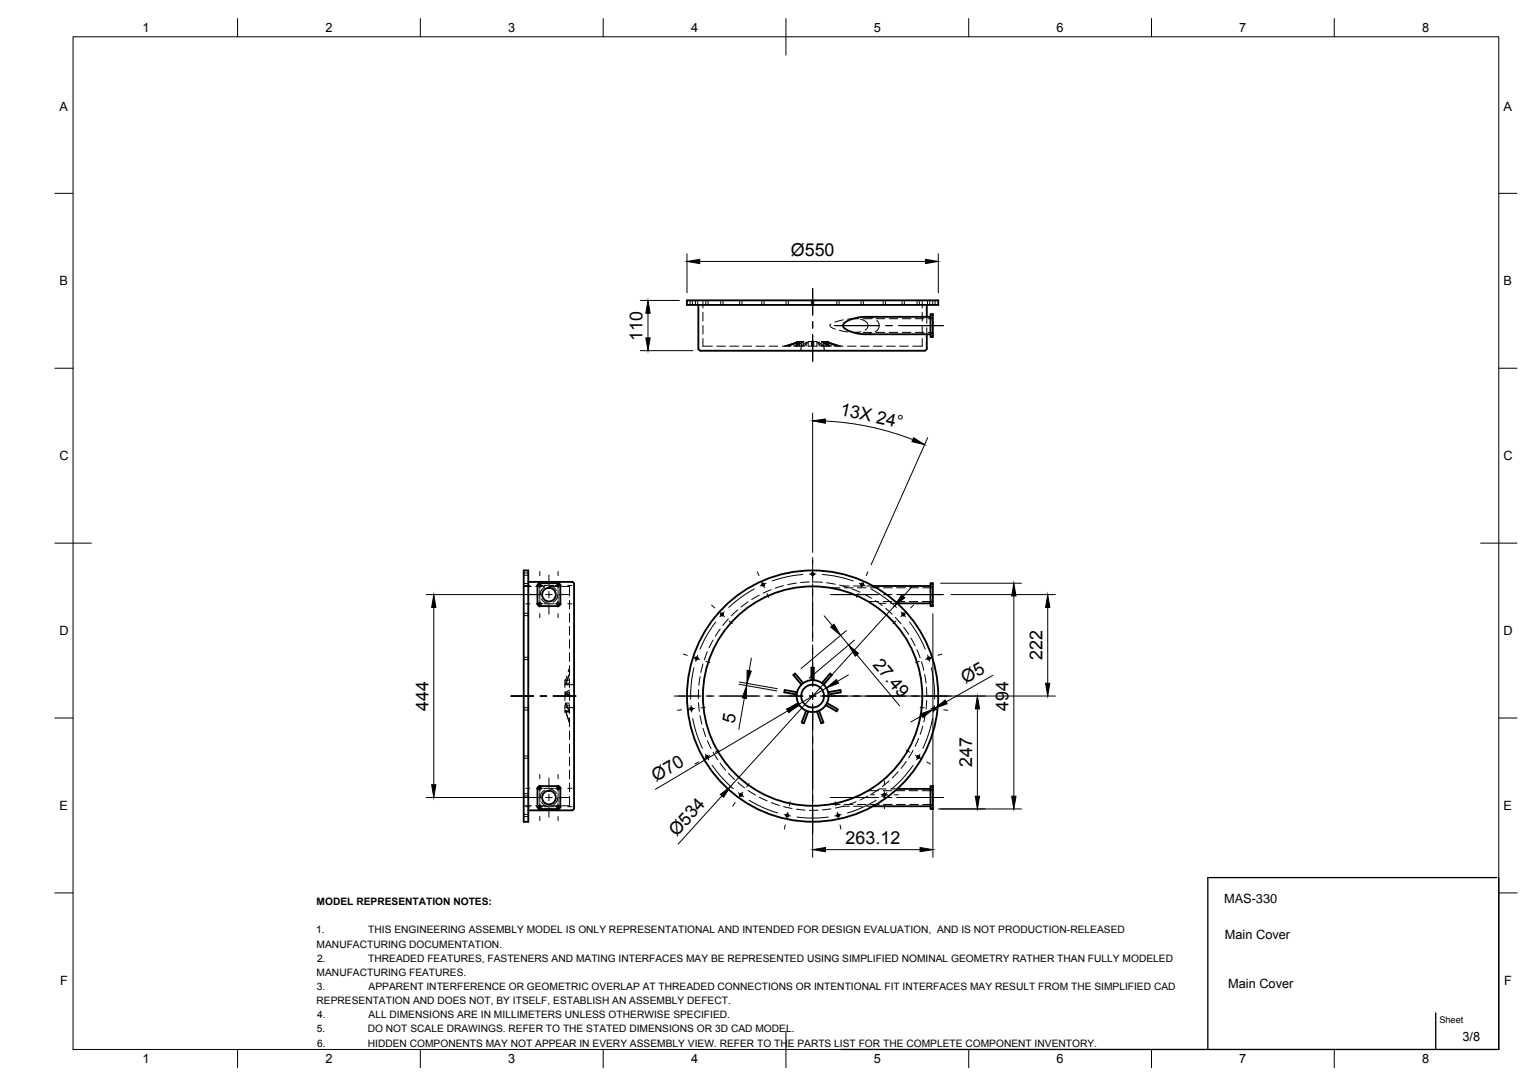
ISO-10303-21;
HEADER;
/* Generated by software containing ST-Developer
 * from STEP Tools, Inc. (www.steptools.com) 
 */

FILE_DESCRIPTION(
/* description */ ('STEP AP214'),
/* implementation_level */ '2;1');

FILE_NAME(
/* name */ 'Main Cover.step',
/* time_stamp */ '2026-10-12T14:05:15-07:00',
/* author */ (''),
/* organization */ (''),
/* preprocessor_version */ 'ST-DEVELOPER v20.2',
/* originating_system */ 'Autodesk Translation Framework v15.15.0.0',
/* authorisation */ '');

FILE_SCHEMA (('AUTOMOTIVE_DESIGN { 1 0 10303 214 3 1 1 }'));
ENDSEC;

DATA;
#10=MECHANICAL_DESIGN_GEOMETRIC_PRESENTATION_REPRESENTATION('',(#282),#39959);
#268=SHAPE_REPRESENTATION_RELATIONSHIP('SRR','None',#40002,#275);
#275=ADVANCED_BREP_SHAPE_REPRESENTATION('',(#290),#39952);
#282=STYLED_ITEM('',(#40046),#290);
#290=MANIFOLD_SOLID_BREP('Body1',#18259);
#297=PLANE('',#18468);
#298=PLANE('',#18469);
#299=PLANE('',#18470);
#300=PLANE('',#18471);
#301=PLANE('',#18472);
#302=PLANE('',#18477);
#303=PLANE('',#18483);
#304=PLANE('',#18485);
#305=PLANE('',#18487);
#306=PLANE('',#18489);
#307=PLANE('',#18490);
#308=PLANE('',#18495);
#309=PLANE('',#18501);
#310=PLANE('',#18503);
#311=PLANE('',#18505);
#312=PLANE('',#18507);
#313=PLANE('',#18508);
#314=PLANE('',#18509);
#315=PLANE('',#18510);
#316=PLANE('',#18511);
#317=PLANE('',#18512);
#318=PLANE('',#18513);
#319=PLANE('',#18514);
#320=PLANE('',#18515);
#321=PLANE('',#18516);
#322=PLANE('',#18517);
#323=PLANE('',#18518);
#324=PLANE('',#18519);
#325=PLANE('',#18520);
#326=PLANE('',#18521);
#327=PLANE('',#18522);
#328=PLANE('',#18523);
#329=PLANE('',#18524);
#330=PLANE('',#18525);
#331=PLANE('',#18526);
#332=PLANE('',#18527);
#333=PLANE('',#18528);
#334=PLANE('',#18529);
#335=PLANE('',#18530);
#336=PLANE('',#18531);
#337=PLANE('',#18532);
#338=PLANE('',#18533);
#339=PLANE('',#18534);
#340=PLANE('',#18535);
#876=FACE_BOUND('',#5847,.T.);
#877=FACE_BOUND('',#5848,.T.);
#878=FACE_BOUND('',#5851,.T.);
#879=FACE_BOUND('',#5852,.T.);
#880=FACE_BOUND('',#5854,.T.);
#881=FACE_BOUND('',#5856,.T.);
#882=FACE_BOUND('',#5857,.T.);
#883=FACE_BOUND('',#5858,.T.);
#884=FACE_BOUND('',#5859,.T.);
#885=FACE_BOUND('',#5860,.T.);
#886=FACE_BOUND('',#5861,.T.);
#887=FACE_BOUND('',#5862,.T.);
#888=FACE_BOUND('',#5863,.T.);
#889=FACE_BOUND('',#5864,.T.);
#890=FACE_BOUND('',#5865,.T.);
#891=FACE_BOUND('',#5866,.T.);
#892=FACE_BOUND('',#5867,.T.);
#893=FACE_BOUND('',#5868,.T.);
#894=FACE_BOUND('',#5869,.T.);
#895=FACE_BOUND('',#5870,.T.);
#896=FACE_BOUND('',#5871,.T.);
#897=FACE_BOUND('',#5873,.T.);
#898=FACE_BOUND('',#5874,.T.);
#899=FACE_BOUND('',#5875,.T.);
#900=FACE_BOUND('',#5876,.T.);
#901=FACE_BOUND('',#5877,.T.);
#902=FACE_BOUND('',#5878,.T.);
#903=FACE_BOUND('',#5879,.T.);
#904=FACE_BOUND('',#5880,.T.);
#905=FACE_BOUND('',#5881,.T.);
#906=FACE_BOUND('',#5882,.T.);
#907=FACE_BOUND('',#5883,.T.);
#908=FACE_BOUND('',#5884,.T.);
#909=FACE_BOUND('',#5885,.T.);
#910=FACE_BOUND('',#5886,.T.);
#911=FACE_BOUND('',#5887,.T.);
#912=FACE_BOUND('',#5888,.T.);
#913=FACE_BOUND('',#5890,.T.);
#914=FACE_BOUND('',#5892,.T.);
#915=FACE_BOUND('',#5893,.T.);
#916=FACE_BOUND('',#5894,.T.);
#917=FACE_BOUND('',#5895,.T.);
#918=FACE_BOUND('',#5896,.T.);
#919=FACE_BOUND('',#5898,.T.);
#920=FACE_BOUND('',#5899,.T.);
#921=FACE_BOUND('',#5900,.T.);
#922=FACE_BOUND('',#5901,.T.);
#923=FACE_BOUND('',#5902,.T.);
#924=FACE_BOUND('',#5912,.T.);
#925=FACE_BOUND('',#5913,.T.);
#926=FACE_BOUND('',#5914,.T.);
#927=FACE_BOUND('',#5915,.T.);
#928=FACE_BOUND('',#5916,.T.);
#929=FACE_BOUND('',#5918,.T.);
#930=FACE_BOUND('',#5919,.T.);
#931=FACE_BOUND('',#5920,.T.);
#932=FACE_BOUND('',#5921,.T.);
#933=FACE_BOUND('',#5922,.T.);
#934=FACE_BOUND('',#5932,.T.);
#1065=B_SPLINE_CURVE_WITH_KNOTS('',3,(#25049,#25050,#25051,#25052,#25053,
#25054,#25055,#25056,#25057,#25058,#25059,#25060,#25061,#25062,#25063,#25064,
#25065,#25066,#25067,#25068,#25069,#25070,#25071,#25072,#25073,#25074,#25075,
#25076,#25077,#25078,#25079,#25080,#25081,#25082,#25083,#25084,#25085,#25086,
#25087,#25088,#25089,#25090,#25091,#25092,#25093,#25094,#25095,#25096,#25097,
#25098,#25099,#25100,#25101,#25102,#25103,#25104,#25105,#25106,#25107,#25108,
#25109,#25110),.UNSPECIFIED.,.T.,.F.,(4,2,2,2,2,2,2,2,2,2,2,2,2,2,2,2,2,
2,2,2,2,2,2,2,2,2,2,2,2,2,4),(-19.6507571622069,-19.4050828429219,-19.1594085236369,
-18.6130728294486,-18.0667371352602,-17.0841171850828,-16.1014972349054,
-15.118877284728,-14.1362573345506,-12.6705405954362,-11.937682225879,-11.2048238563218,
-10.8599625375172,-10.5151012187126,-10.170239899908,-9.82537858110344,
-9.48051726229887,-9.13565594349429,-8.79079462468971,-8.44593330588513,
-7.71307493632793,-6.98021656677073,-5.51449982765633,-4.53187987747891,
-3.54925992730149,-2.56663997712407,-1.58402002694665,-1.03768433275833,
-0.491348638570005,-0.245674319285003,0.),.UNSPECIFIED.);
#1066=B_SPLINE_CURVE_WITH_KNOTS('',3,(#25116,#25117,#25118,#25119,#25120,
#25121,#25122,#25123,#25124,#25125,#25126,#25127,#25128,#25129,#25130,#25131,
#25132,#25133,#25134,#25135,#25136,#25137,#25138,#25139,#25140,#25141,#25142,
#25143,#25144,#25145,#25146,#25147,#25148,#25149,#25150,#25151,#25152,#25153,
#25154,#25155,#25156,#25157,#25158,#25159,#25160,#25161,#25162,#25163,#25164,
#25165,#25166,#25167,#25168,#25169,#25170,#25171,#25172,#25173,#25174,#25175,
#25176,#25177),.UNSPECIFIED.,.T.,.F.,(4,2,2,2,2,2,2,2,2,2,2,2,2,2,2,2,2,
2,2,2,2,2,2,2,2,2,2,2,2,2,4),(-19.6507571622069,-19.3058958434024,-18.9610345245978,
-18.6161732057932,-18.2713118869886,-17.5384535174314,-16.8055951478742,
-15.3398784087598,-14.3572584585824,-13.374638508405,-12.3920185582275,
-11.4093986080501,-10.8630629138618,-10.3167272196735,-10.0710529003885,
-9.82537858110347,-9.57970426181847,-9.33402994253347,-8.78769424834514,
-8.24135855415682,-7.25873860397939,-6.27611865380197,-5.29349870362454,
-4.31087875344711,-2.84516201433271,-2.11230364477551,-1.37944527521831,
-1.03458395641373,-0.689722637609155,-0.344861318804578,0.),
 .UNSPECIFIED.);
#1067=B_SPLINE_CURVE_WITH_KNOTS('',3,(#25183,#25184,#25185,#25186,#25187,
#25188,#25189,#25190,#25191,#25192,#25193,#25194,#25195,#25196,#25197,#25198,
#25199,#25200,#25201,#25202,#25203,#25204,#25205,#25206,#25207,#25208,#25209,
#25210,#25211,#25212,#25213,#25214,#25215,#25216,#25217,#25218,#25219,#25220,
#25221,#25222,#25223,#25224,#25225,#25226,#25227,#25228,#25229,#25230,#25231,
#25232,#25233,#25234,#25235,#25236,#25237,#25238,#25239,#25240,#25241,#25242,
#25243,#25244,#25245,#25246,#25247,#25248),.UNSPECIFIED.,.T.,.F.,(4,2,2,
2,2,2,2,2,2,2,2,2,2,2,2,2,2,2,2,2,2,2,2,2,2,2,2,2,2,2,2,2,4),(-18.9027433334398,
-18.6305373935122,-18.3583314535845,-17.8139195737293,-17.1230429609855,
-16.4321663482417,-15.050413122754,-14.0219604634627,-12.9935078041713,
-11.9650551448799,-10.9366024855886,-10.3754064287965,-10.0948084004005,
-9.81421037200448,-9.63279101936218,-9.54208134304104,-9.45137166671989,
-9.36066199039874,-9.26995231407759,-9.08853296143529,-8.80793493303927,
-8.52733690464326,-7.96614084785122,-6.93768818855985,-5.90923552926848,
-4.88078286997711,-3.85233021068574,-2.47057698519811,-1.7797003724543,
-1.08882375971048,-0.54441187985524,-0.27220593992762,0.),.UNSPECIFIED.);
#1068=B_SPLINE_CURVE_WITH_KNOTS('',3,(#25254,#25255,#25256,#25257,#25258,
#25259,#25260,#25261,#25262,#25263,#25264,#25265,#25266,#25267,#25268,#25269,
#25270,#25271,#25272,#25273,#25274,#25275,#25276,#25277,#25278,#25279,#25280,
#25281,#25282,#25283,#25284,#25285,#25286,#25287,#25288,#25289,#25290,#25291,
#25292,#25293,#25294,#25295,#25296,#25297,#25298,#25299,#25300,#25301,#25302,
#25303,#25304,#25305,#25306,#25307,#25308,#25309,#25310,#25311,#25312,#25313,
#25314,#25315,#25316,#25317,#25318,#25319),.UNSPECIFIED.,.T.,.F.,(4,2,2,
2,2,2,2,2,2,2,2,2,2,2,2,2,2,2,2,2,2,2,2,2,2,2,2,2,2,2,2,2,4),(-18.9027433334398,
-18.8120336571186,-18.7213239807975,-18.5399046281552,-18.2593065997592,
-17.9787085713631,-17.4175125145711,-16.3890598552797,-15.3606071959884,
-14.332154536697,-13.3037018774056,-11.921948651918,-11.2310720391742,-10.5401954264304,
-9.99578354657513,-9.72357760664751,-9.45137166671989,-9.17916572679227,
-8.90695978686465,-8.36254790700941,-7.67167129426559,-6.98079468152178,
-5.59904145603415,-4.57058879674278,-3.54213613745141,-2.51368347816004,
-1.48523081886867,-0.924034762076629,-0.643436733680611,-0.362838705284593,
-0.181419352642297,-0.0907096763211483,0.),.UNSPECIFIED.);
#1368=ELLIPSE('',#18362,36.6292398804354,35.);
#1369=ELLIPSE('',#18364,36.6292398804354,35.);
#1370=ELLIPSE('',#18366,36.6292398804354,35.);
#1371=ELLIPSE('',#18368,36.6292398804354,35.);
#1372=ELLIPSE('',#18372,36.6292398804354,35.);
#1373=ELLIPSE('',#18374,36.6292398804354,35.);
#1374=ELLIPSE('',#18376,36.6292398804354,35.);
#1375=ELLIPSE('',#18378,36.6292398804354,35.);
#1376=ELLIPSE('',#18380,36.6292398804354,35.);
#1408=LINE('',#24926,#2981);
#1409=LINE('',#24930,#2982);
#1410=LINE('',#24934,#2983);
#1411=LINE('',#24938,#2984);
#1412=LINE('',#24942,#2985);
#1413=LINE('',#24946,#2986);
#1414=LINE('',#24950,#2987);
#1415=LINE('',#24954,#2988);
#1416=LINE('',#24958,#2989);
#1417=LINE('',#24963,#2990);
#1418=LINE('',#24967,#2991);
#1419=LINE('',#24971,#2992);
#1420=LINE('',#24975,#2993);
#1421=LINE('',#24979,#2994);
#1422=LINE('',#24983,#2995);
#1423=LINE('',#24987,#2996);
#1424=LINE('',#24991,#2997);
#1425=LINE('',#24995,#2998);
#1426=LINE('',#24998,#2999);
#1427=LINE('',#25003,#3000);
#1428=LINE('',#25009,#3001);
#1429=LINE('',#25015,#3002);
#1430=LINE('',#25021,#3003);
#1431=LINE('',#25027,#3004);
#1432=LINE('',#25033,#3005);
#1433=LINE('',#25039,#3006);
#1434=LINE('',#25045,#3007);
#1435=LINE('',#25112,#3008);
#1436=LINE('',#25179,#3009);
#1437=LINE('',#25250,#3010);
#1438=LINE('',#25321,#3011);
#1439=LINE('',#25325,#3012);
#1440=LINE('',#25331,#3013);
#1441=LINE('',#25337,#3014);
#1442=LINE('',#25343,#3015);
#1443=LINE('',#25349,#3016);
#1444=LINE('',#25355,#3017);
#1445=LINE('',#25361,#3018);
#1446=LINE('',#25367,#3019);
#1447=LINE('',#25373,#3020);
#1448=LINE('',#25379,#3021);
#1449=LINE('',#25385,#3022);
#1450=LINE('',#25391,#3023);
#1451=LINE('',#25397,#3024);
#1452=LINE('',#25403,#3025);
#1453=LINE('',#25409,#3026);
#1454=LINE('',#25415,#3027);
#1455=LINE('',#25419,#3028);
#1456=LINE('',#25425,#3029);
#1457=LINE('',#25431,#3030);
#1458=LINE('',#25435,#3031);
#1459=LINE('',#25437,#3032);
#1460=LINE('',#25439,#3033);
#1461=LINE('',#25440,#3034);
#1462=LINE('',#25442,#3035);
#1463=LINE('',#25444,#3036);
#1464=LINE('',#25445,#3037);
#1465=LINE('',#25447,#3038);
#1466=LINE('',#25449,#3039);
#1467=LINE('',#25450,#3040);
#1468=LINE('',#25452,#3041);
#1469=LINE('',#25454,#3042);
#1470=LINE('',#25455,#3043);
#1471=LINE('',#25457,#3044);
#1472=LINE('',#25459,#3045);
#1473=LINE('',#25460,#3046);
#1474=LINE('',#25462,#3047);
#1475=LINE('',#25464,#3048);
#1476=LINE('',#25465,#3049);
#1477=LINE('',#25467,#3050);
#1478=LINE('',#25469,#3051);
#1479=LINE('',#25470,#3052);
#1480=LINE('',#25472,#3053);
#1481=LINE('',#25474,#3054);
#1482=LINE('',#25475,#3055);
#1483=LINE('',#25477,#3056);
#1484=LINE('',#25478,#3057);
#1485=LINE('',#25487,#3058);
#1486=LINE('',#25491,#3059);
#1487=LINE('',#25495,#3060);
#1488=LINE('',#25498,#3061);
#1489=LINE('',#25504,#3062);
#1490=LINE('',#25508,#3063);
#1491=LINE('',#25512,#3064);
#1492=LINE('',#25515,#3065);
#1493=LINE('',#25517,#3066);
#1494=LINE('',#25518,#3067);
#1495=LINE('',#25520,#3068);
#1496=LINE('',#25522,#3069);
#1497=LINE('',#25524,#3070);
#1498=LINE('',#25526,#3071);
#1499=LINE('',#25528,#3072);
#1500=LINE('',#25530,#3073);
#1501=LINE('',#25537,#3074);
#1502=LINE('',#25541,#3075);
#1503=LINE('',#25545,#3076);
#1504=LINE('',#25548,#3077);
#1505=LINE('',#25554,#3078);
#1506=LINE('',#25558,#3079);
#1507=LINE('',#25562,#3080);
#1508=LINE('',#25565,#3081);
#1509=LINE('',#25567,#3082);
#1510=LINE('',#25568,#3083);
#1511=LINE('',#25570,#3084);
#1512=LINE('',#25572,#3085);
#1513=LINE('',#25574,#3086);
#1514=LINE('',#25576,#3087);
#1515=LINE('',#25578,#3088);
#1516=LINE('',#25580,#3089);
#1517=LINE('',#25584,#3090);
#1518=LINE('',#25586,#3091);
#1519=LINE('',#25589,#3092);
#1520=LINE('',#25591,#3093);
#1521=LINE('',#25594,#3094);
#1522=LINE('',#25596,#3095);
#1523=LINE('',#25599,#3096);
#1524=LINE('',#25601,#3097);
#1525=LINE('',#25604,#3098);
#1526=LINE('',#25606,#3099);
#1527=LINE('',#25609,#3100);
#1528=LINE('',#25611,#3101);
#1529=LINE('',#25614,#3102);
#1530=LINE('',#25616,#3103);
#1531=LINE('',#25619,#3104);
#1532=LINE('',#25621,#3105);
#1533=LINE('',#25624,#3106);
#1534=LINE('',#25626,#3107);
#2981=VECTOR('',#20036,1000.);
#2982=VECTOR('',#20039,1000.);
#2983=VECTOR('',#20042,1000.);
#2984=VECTOR('',#20045,1000.);
#2985=VECTOR('',#20048,1000.);
#2986=VECTOR('',#20051,1000.);
#2987=VECTOR('',#20054,1000.);
#2988=VECTOR('',#20057,1000.);
#2989=VECTOR('',#20060,35.);
#2990=VECTOR('',#20065,1000.);
#2991=VECTOR('',#20068,1000.);
#2992=VECTOR('',#20071,1000.);
#2993=VECTOR('',#20074,1000.);
#2994=VECTOR('',#20077,1000.);
#2995=VECTOR('',#20080,1000.);
#2996=VECTOR('',#20083,1000.);
#2997=VECTOR('',#20086,1000.);
#2998=VECTOR('',#20089,1000.);
#2999=VECTOR('',#20092,1000.);
#3000=VECTOR('',#20097,2.5);
#3001=VECTOR('',#20104,2.49999999999997);
#3002=VECTOR('',#20111,2.5);
#3003=VECTOR('',#20118,2.5);
#3004=VECTOR('',#20125,2.49999999999997);
#3005=VECTOR('',#20132,2.5);
#3006=VECTOR('',#20139,2.5);
#3007=VECTOR('',#20146,2.5);
#3008=VECTOR('',#20151,19.);
#3009=VECTOR('',#20156,19.);
#3010=VECTOR('',#20161,15.);
#3011=VECTOR('',#20166,15.);
#3012=VECTOR('',#20171,25.);
#3013=VECTOR('',#20178,2.5);
#3014=VECTOR('',#20185,2.5);
#3015=VECTOR('',#20192,2.5);
#3016=VECTOR('',#20199,2.5);
#3017=VECTOR('',#20206,2.5);
#3018=VECTOR('',#20213,2.5);
#3019=VECTOR('',#20220,2.5);
#3020=VECTOR('',#20227,2.5);
#3021=VECTOR('',#20234,2.50000000000001);
#3022=VECTOR('',#20241,2.5);
#3023=VECTOR('',#20248,2.5);
#3024=VECTOR('',#20255,2.5);
#3025=VECTOR('',#20262,2.5);
#3026=VECTOR('',#20269,2.5);
#3027=VECTOR('',#20276,2.5);
#3028=VECTOR('',#20281,250.);
#3029=VECTOR('',#20288,275.);
#3030=VECTOR('',#20295,240.);
#3031=VECTOR('',#20300,1000.);
#3032=VECTOR('',#20301,1000.);
#3033=VECTOR('',#20302,1000.);
#3034=VECTOR('',#20303,1000.);
#3035=VECTOR('',#20304,1000.);
#3036=VECTOR('',#20305,1000.);
#3037=VECTOR('',#20306,1000.);
#3038=VECTOR('',#20307,1000.);
#3039=VECTOR('',#20308,1000.);
#3040=VECTOR('',#20309,1000.);
#3041=VECTOR('',#20310,1000.);
#3042=VECTOR('',#20311,1000.);
#3043=VECTOR('',#20312,1000.);
#3044=VECTOR('',#20313,1000.);
#3045=VECTOR('',#20314,1000.);
#3046=VECTOR('',#20315,1000.);
#3047=VECTOR('',#20316,1000.);
#3048=VECTOR('',#20317,1000.);
#3049=VECTOR('',#20318,1000.);
#3050=VECTOR('',#20319,1000.);
#3051=VECTOR('',#20320,1000.);
#3052=VECTOR('',#20321,1000.);
#3053=VECTOR('',#20322,1000.);
#3054=VECTOR('',#20323,1000.);
#3055=VECTOR('',#20324,1000.);
#3056=VECTOR('',#20325,1000.);
#3057=VECTOR('',#20326,1000.);
#3058=VECTOR('',#20337,1000.);
#3059=VECTOR('',#20340,1000.);
#3060=VECTOR('',#20343,1000.);
#3061=VECTOR('',#20346,1000.);
#3062=VECTOR('',#20351,1000.);
#3063=VECTOR('',#20354,1000.);
#3064=VECTOR('',#20357,1000.);
#3065=VECTOR('',#20360,1000.);
#3066=VECTOR('',#20363,1000.);
#3067=VECTOR('',#20364,1000.);
#3068=VECTOR('',#20367,1000.);
#3069=VECTOR('',#20370,1000.);
#3070=VECTOR('',#20373,1000.);
#3071=VECTOR('',#20376,1000.);
#3072=VECTOR('',#20379,1000.);
#3073=VECTOR('',#20382,1000.);
#3074=VECTOR('',#20389,1000.);
#3075=VECTOR('',#20392,1000.);
#3076=VECTOR('',#20395,1000.);
#3077=VECTOR('',#20398,1000.);
#3078=VECTOR('',#20403,1000.);
#3079=VECTOR('',#20406,1000.);
#3080=VECTOR('',#20409,1000.);
#3081=VECTOR('',#20412,1000.);
#3082=VECTOR('',#20415,1000.);
#3083=VECTOR('',#20416,1000.);
#3084=VECTOR('',#20419,1000.);
#3085=VECTOR('',#20422,1000.);
#3086=VECTOR('',#20425,1000.);
#3087=VECTOR('',#20428,1000.);
#3088=VECTOR('',#20431,1000.);
#3089=VECTOR('',#20434,1000.);
#3090=VECTOR('',#20441,1000.);
#3091=VECTOR('',#20444,1000.);
#3092=VECTOR('',#20449,1000.);
#3093=VECTOR('',#20452,1000.);
#3094=VECTOR('',#20457,1000.);
#3095=VECTOR('',#20460,1000.);
#3096=VECTOR('',#20465,1000.);
#3097=VECTOR('',#20468,1000.);
#3098=VECTOR('',#20473,1000.);
#3099=VECTOR('',#20476,1000.);
#3100=VECTOR('',#20481,1000.);
#3101=VECTOR('',#20484,1000.);
#3102=VECTOR('',#20489,1000.);
#3103=VECTOR('',#20492,1000.);
#3104=VECTOR('',#20497,1000.);
#3105=VECTOR('',#20500,1000.);
#3106=VECTOR('',#20505,1000.);
#3107=VECTOR('',#20508,1000.);
#4554=CYLINDRICAL_SURFACE('',#18360,35.);
#4555=CYLINDRICAL_SURFACE('',#18381,2.5);
#4556=CYLINDRICAL_SURFACE('',#18384,2.49999999999997);
#4557=CYLINDRICAL_SURFACE('',#18387,2.5);
#4558=CYLINDRICAL_SURFACE('',#18390,2.5);
#4559=CYLINDRICAL_SURFACE('',#18393,2.49999999999997);
#4560=CYLINDRICAL_SURFACE('',#18396,2.5);
#4561=CYLINDRICAL_SURFACE('',#18399,2.5);
#4562=CYLINDRICAL_SURFACE('',#18402,2.5);
#4563=CYLINDRICAL_SURFACE('',#18405,19.);
#4564=CYLINDRICAL_SURFACE('',#18407,19.);
#4565=CYLINDRICAL_SURFACE('',#18409,15.);
#4566=CYLINDRICAL_SURFACE('',#18411,15.);
#4567=CYLINDRICAL_SURFACE('',#18413,25.);
#4568=CYLINDRICAL_SURFACE('',#18415,2.5);
#4569=CYLINDRICAL_SURFACE('',#18418,2.5);
#4570=CYLINDRICAL_SURFACE('',#18421,2.5);
#4571=CYLINDRICAL_SURFACE('',#18424,2.5);
#4572=CYLINDRICAL_SURFACE('',#18427,2.5);
#4573=CYLINDRICAL_SURFACE('',#18430,2.5);
#4574=CYLINDRICAL_SURFACE('',#18433,2.5);
#4575=CYLINDRICAL_SURFACE('',#18436,2.5);
#4576=CYLINDRICAL_SURFACE('',#18439,2.50000000000001);
#4577=CYLINDRICAL_SURFACE('',#18442,2.5);
#4578=CYLINDRICAL_SURFACE('',#18445,2.5);
#4579=CYLINDRICAL_SURFACE('',#18448,2.5);
#4580=CYLINDRICAL_SURFACE('',#18451,2.5);
#4581=CYLINDRICAL_SURFACE('',#18454,2.5);
#4582=CYLINDRICAL_SURFACE('',#18457,2.5);
#4583=CYLINDRICAL_SURFACE('',#18460,250.);
#4584=CYLINDRICAL_SURFACE('',#18462,275.);
#4585=CYLINDRICAL_SURFACE('',#18465,240.);
#4586=CYLINDRICAL_SURFACE('',#18482,5.);
#4587=CYLINDRICAL_SURFACE('',#18484,5.);
#4588=CYLINDRICAL_SURFACE('',#18486,5.00000000000003);
#4589=CYLINDRICAL_SURFACE('',#18488,5.);
#4590=CYLINDRICAL_SURFACE('',#18500,5.);
#4591=CYLINDRICAL_SURFACE('',#18502,5.);
#4592=CYLINDRICAL_SURFACE('',#18504,5.);
#4593=CYLINDRICAL_SURFACE('',#18506,5.00000000000003);
#4822=FACE_OUTER_BOUND('',#5815,.T.);
#4823=FACE_OUTER_BOUND('',#5816,.T.);
#4824=FACE_OUTER_BOUND('',#5817,.T.);
#4825=FACE_OUTER_BOUND('',#5818,.T.);
#4826=FACE_OUTER_BOUND('',#5819,.T.);
#4827=FACE_OUTER_BOUND('',#5820,.T.);
#4828=FACE_OUTER_BOUND('',#5821,.T.);
#4829=FACE_OUTER_BOUND('',#5822,.T.);
#4830=FACE_OUTER_BOUND('',#5823,.T.);
#4831=FACE_OUTER_BOUND('',#5824,.T.);
#4832=FACE_OUTER_BOUND('',#5825,.T.);
#4833=FACE_OUTER_BOUND('',#5826,.T.);
#4834=FACE_OUTER_BOUND('',#5827,.T.);
#4835=FACE_OUTER_BOUND('',#5828,.T.);
#4836=FACE_OUTER_BOUND('',#5829,.T.);
#4837=FACE_OUTER_BOUND('',#5830,.T.);
#4838=FACE_OUTER_BOUND('',#5831,.T.);
#4839=FACE_OUTER_BOUND('',#5832,.T.);
#4840=FACE_OUTER_BOUND('',#5833,.T.);
#4841=FACE_OUTER_BOUND('',#5834,.T.);
#4842=FACE_OUTER_BOUND('',#5835,.T.);
#4843=FACE_OUTER_BOUND('',#5836,.T.);
#4844=FACE_OUTER_BOUND('',#5837,.T.);
#4845=FACE_OUTER_BOUND('',#5838,.T.);
#4846=FACE_OUTER_BOUND('',#5839,.T.);
#4847=FACE_OUTER_BOUND('',#5840,.T.);
#4848=FACE_OUTER_BOUND('',#5841,.T.);
#4849=FACE_OUTER_BOUND('',#5842,.T.);
#4850=FACE_OUTER_BOUND('',#5843,.T.);
#4851=FACE_OUTER_BOUND('',#5844,.T.);
#4852=FACE_OUTER_BOUND('',#5845,.T.);
#4853=FACE_OUTER_BOUND('',#5846,.T.);
#4854=FACE_OUTER_BOUND('',#5849,.T.);
#4855=FACE_OUTER_BOUND('',#5850,.T.);
#4856=FACE_OUTER_BOUND('',#5853,.T.);
#4857=FACE_OUTER_BOUND('',#5855,.T.);
#4858=FACE_OUTER_BOUND('',#5872,.T.);
#4859=FACE_OUTER_BOUND('',#5889,.T.);
#4860=FACE_OUTER_BOUND('',#5891,.T.);
#4861=FACE_OUTER_BOUND('',#5897,.T.);
#4862=FACE_OUTER_BOUND('',#5903,.T.);
#4863=FACE_OUTER_BOUND('',#5904,.T.);
#4864=FACE_OUTER_BOUND('',#5905,.T.);
#4865=FACE_OUTER_BOUND('',#5906,.T.);
#4866=FACE_OUTER_BOUND('',#5907,.T.);
#4867=FACE_OUTER_BOUND('',#5908,.T.);
#4868=FACE_OUTER_BOUND('',#5909,.T.);
#4869=FACE_OUTER_BOUND('',#5910,.T.);
#4870=FACE_OUTER_BOUND('',#5911,.T.);
#4871=FACE_OUTER_BOUND('',#5917,.T.);
#4872=FACE_OUTER_BOUND('',#5923,.T.);
#4873=FACE_OUTER_BOUND('',#5924,.T.);
#4874=FACE_OUTER_BOUND('',#5925,.T.);
#4875=FACE_OUTER_BOUND('',#5926,.T.);
#4876=FACE_OUTER_BOUND('',#5927,.T.);
#4877=FACE_OUTER_BOUND('',#5928,.T.);
#4878=FACE_OUTER_BOUND('',#5929,.T.);
#4879=FACE_OUTER_BOUND('',#5930,.T.);
#4880=FACE_OUTER_BOUND('',#5931,.T.);
#4881=FACE_OUTER_BOUND('',#5933,.T.);
#4882=FACE_OUTER_BOUND('',#5934,.T.);
#4883=FACE_OUTER_BOUND('',#5935,.T.);
#4884=FACE_OUTER_BOUND('',#5936,.T.);
#4885=FACE_OUTER_BOUND('',#5937,.T.);
#4886=FACE_OUTER_BOUND('',#5938,.T.);
#4887=FACE_OUTER_BOUND('',#5939,.T.);
#4888=FACE_OUTER_BOUND('',#5940,.T.);
#4889=FACE_OUTER_BOUND('',#5941,.T.);
#4890=FACE_OUTER_BOUND('',#5942,.T.);
#4891=FACE_OUTER_BOUND('',#5943,.T.);
#4892=FACE_OUTER_BOUND('',#5944,.T.);
#4893=FACE_OUTER_BOUND('',#5945,.T.);
#4894=FACE_OUTER_BOUND('',#5946,.T.);
#4895=FACE_OUTER_BOUND('',#5947,.T.);
#4896=FACE_OUTER_BOUND('',#5948,.T.);
#4897=FACE_OUTER_BOUND('',#5949,.T.);
#4898=FACE_OUTER_BOUND('',#5950,.T.);
#4899=FACE_OUTER_BOUND('',#5951,.T.);
#4900=FACE_OUTER_BOUND('',#5952,.T.);
#4901=FACE_OUTER_BOUND('',#5953,.T.);
#4902=FACE_OUTER_BOUND('',#5954,.T.);
#4903=FACE_OUTER_BOUND('',#5955,.T.);
#4904=FACE_OUTER_BOUND('',#5956,.T.);
#4905=FACE_OUTER_BOUND('',#5957,.T.);
#4906=FACE_OUTER_BOUND('',#5958,.T.);
#4907=FACE_OUTER_BOUND('',#5959,.T.);
#5815=EDGE_LOOP('',(#12006,#12007,#12008,#12009));
#5816=EDGE_LOOP('',(#12010,#12011,#12012,#12013,#12014));
#5817=EDGE_LOOP('',(#12015,#12016,#12017,#12018,#12019,#12020,#12021,#12022,
#12023,#12024,#12025,#12026,#12027,#12028,#12029,#12030,#12031,#12032,#12033,
#12034,#12035,#12036,#12037,#12038,#12039,#12040,#12041,#12042,#12043,#12044,
#12045,#12046,#12047,#12048,#12049,#12050,#12051,#12052,#12053,#12054));
#5818=EDGE_LOOP('',(#12055,#12056,#12057,#12058));
#5819=EDGE_LOOP('',(#12059,#12060,#12061,#12062));
#5820=EDGE_LOOP('',(#12063,#12064,#12065,#12066));
#5821=EDGE_LOOP('',(#12067,#12068,#12069,#12070));
#5822=EDGE_LOOP('',(#12071,#12072,#12073,#12074));
#5823=EDGE_LOOP('',(#12075,#12076,#12077,#12078));
#5824=EDGE_LOOP('',(#12079,#12080,#12081,#12082));
#5825=EDGE_LOOP('',(#12083,#12084,#12085,#12086));
#5826=EDGE_LOOP('',(#12087,#12088,#12089,#12090));
#5827=EDGE_LOOP('',(#12091,#12092,#12093,#12094));
#5828=EDGE_LOOP('',(#12095,#12096,#12097,#12098));
#5829=EDGE_LOOP('',(#12099,#12100,#12101,#12102));
#5830=EDGE_LOOP('',(#12103,#12104,#12105,#12106));
#5831=EDGE_LOOP('',(#12107,#12108,#12109,#12110));
#5832=EDGE_LOOP('',(#12111,#12112,#12113,#12114));
#5833=EDGE_LOOP('',(#12115,#12116,#12117,#12118));
#5834=EDGE_LOOP('',(#12119,#12120,#12121,#12122));
#5835=EDGE_LOOP('',(#12123,#12124,#12125,#12126));
#5836=EDGE_LOOP('',(#12127,#12128,#12129,#12130));
#5837=EDGE_LOOP('',(#12131,#12132,#12133,#12134));
#5838=EDGE_LOOP('',(#12135,#12136,#12137,#12138));
#5839=EDGE_LOOP('',(#12139,#12140,#12141,#12142));
#5840=EDGE_LOOP('',(#12143,#12144,#12145,#12146));
#5841=EDGE_LOOP('',(#12147,#12148,#12149,#12150));
#5842=EDGE_LOOP('',(#12151,#12152,#12153,#12154));
#5843=EDGE_LOOP('',(#12155,#12156,#12157,#12158));
#5844=EDGE_LOOP('',(#12159,#12160,#12161,#12162));
#5845=EDGE_LOOP('',(#12163,#12164,#12165,#12166));
#5846=EDGE_LOOP('',(#12167,#12168,#12169,#12170,#12171));
#5847=EDGE_LOOP('',(#12172));
#5848=EDGE_LOOP('',(#12173));
#5849=EDGE_LOOP('',(#12174,#12175,#12176,#12177));
#5850=EDGE_LOOP('',(#12178,#12179,#12180,#12181));
#5851=EDGE_LOOP('',(#12182));
#5852=EDGE_LOOP('',(#12183));
#5853=EDGE_LOOP('',(#12184));
#5854=EDGE_LOOP('',(#12185,#12186,#12187,#12188,#12189,#12190,#12191,#12192,
#12193,#12194,#12195,#12196,#12197,#12198,#12199,#12200,#12201,#12202,#12203,
#12204,#12205,#12206,#12207,#12208,#12209,#12210,#12211,#12212,#12213,#12214,
#12215,#12216,#12217,#12218,#12219,#12220,#12221));
#5855=EDGE_LOOP('',(#12222));
#5856=EDGE_LOOP('',(#12223));
#5857=EDGE_LOOP('',(#12224));
#5858=EDGE_LOOP('',(#12225));
#5859=EDGE_LOOP('',(#12226));
#5860=EDGE_LOOP('',(#12227));
#5861=EDGE_LOOP('',(#12228));
#5862=EDGE_LOOP('',(#12229));
#5863=EDGE_LOOP('',(#12230));
#5864=EDGE_LOOP('',(#12231));
#5865=EDGE_LOOP('',(#12232));
#5866=EDGE_LOOP('',(#12233));
#5867=EDGE_LOOP('',(#12234));
#5868=EDGE_LOOP('',(#12235));
#5869=EDGE_LOOP('',(#12236));
#5870=EDGE_LOOP('',(#12237));
#5871=EDGE_LOOP('',(#12238));
#5872=EDGE_LOOP('',(#12239));
#5873=EDGE_LOOP('',(#12240));
#5874=EDGE_LOOP('',(#12241));
#5875=EDGE_LOOP('',(#12242));
#5876=EDGE_LOOP('',(#12243));
#5877=EDGE_LOOP('',(#12244));
#5878=EDGE_LOOP('',(#12245));
#5879=EDGE_LOOP('',(#12246));
#5880=EDGE_LOOP('',(#12247));
#5881=EDGE_LOOP('',(#12248));
#5882=EDGE_LOOP('',(#12249));
#5883=EDGE_LOOP('',(#12250));
#5884=EDGE_LOOP('',(#12251));
#5885=EDGE_LOOP('',(#12252));
#5886=EDGE_LOOP('',(#12253));
#5887=EDGE_LOOP('',(#12254));
#5888=EDGE_LOOP('',(#12255));
#5889=EDGE_LOOP('',(#12256));
#5890=EDGE_LOOP('',(#12257));
#5891=EDGE_LOOP('',(#12258,#12259,#12260,#12261,#12262,#12263,#12264,#12265));
#5892=EDGE_LOOP('',(#12266));
#5893=EDGE_LOOP('',(#12267));
#5894=EDGE_LOOP('',(#12268));
#5895=EDGE_LOOP('',(#12269));
#5896=EDGE_LOOP('',(#12270));
#5897=EDGE_LOOP('',(#12271,#12272,#12273,#12274,#12275,#12276,#12277,#12278));
#5898=EDGE_LOOP('',(#12279));
#5899=EDGE_LOOP('',(#12280));
#5900=EDGE_LOOP('',(#12281));
#5901=EDGE_LOOP('',(#12282));
#5902=EDGE_LOOP('',(#12283));
#5903=EDGE_LOOP('',(#12284,#12285,#12286,#12287));
#5904=EDGE_LOOP('',(#12288,#12289,#12290,#12291));
#5905=EDGE_LOOP('',(#12292,#12293,#12294,#12295));
#5906=EDGE_LOOP('',(#12296,#12297,#12298,#12299));
#5907=EDGE_LOOP('',(#12300,#12301,#12302,#12303));
#5908=EDGE_LOOP('',(#12304,#12305,#12306,#12307));
#5909=EDGE_LOOP('',(#12308,#12309,#12310,#12311));
#5910=EDGE_LOOP('',(#12312,#12313,#12314,#12315));
#5911=EDGE_LOOP('',(#12316,#12317,#12318,#12319,#12320,#12321,#12322,#12323));
#5912=EDGE_LOOP('',(#12324));
#5913=EDGE_LOOP('',(#12325));
#5914=EDGE_LOOP('',(#12326));
#5915=EDGE_LOOP('',(#12327));
#5916=EDGE_LOOP('',(#12328));
#5917=EDGE_LOOP('',(#12329,#12330,#12331,#12332,#12333,#12334,#12335,#12336));
#5918=EDGE_LOOP('',(#12337));
#5919=EDGE_LOOP('',(#12338));
#5920=EDGE_LOOP('',(#12339));
#5921=EDGE_LOOP('',(#12340));
#5922=EDGE_LOOP('',(#12341));
#5923=EDGE_LOOP('',(#12342,#12343,#12344,#12345));
#5924=EDGE_LOOP('',(#12346,#12347,#12348,#12349));
#5925=EDGE_LOOP('',(#12350,#12351,#12352,#12353));
#5926=EDGE_LOOP('',(#12354,#12355,#12356,#12357));
#5927=EDGE_LOOP('',(#12358,#12359,#12360,#12361));
#5928=EDGE_LOOP('',(#12362,#12363,#12364,#12365));
#5929=EDGE_LOOP('',(#12366,#12367,#12368,#12369));
#5930=EDGE_LOOP('',(#12370,#12371,#12372,#12373));
#5931=EDGE_LOOP('',(#12374));
#5932=EDGE_LOOP('',(#12375));
#5933=EDGE_LOOP('',(#12376,#12377,#12378));
#5934=EDGE_LOOP('',(#12379,#12380,#12381));
#5935=EDGE_LOOP('',(#12382,#12383,#12384,#12385));
#5936=EDGE_LOOP('',(#12386,#12387,#12388));
#5937=EDGE_LOOP('',(#12389,#12390,#12391));
#5938=EDGE_LOOP('',(#12392,#12393,#12394,#12395));
#5939=EDGE_LOOP('',(#12396,#12397,#12398));
#5940=EDGE_LOOP('',(#12399,#12400,#12401));
#5941=EDGE_LOOP('',(#12402,#12403,#12404,#12405));
#5942=EDGE_LOOP('',(#12406,#12407,#12408));
#5943=EDGE_LOOP('',(#12409,#12410,#12411));
#5944=EDGE_LOOP('',(#12412,#12413,#12414,#12415));
#5945=EDGE_LOOP('',(#12416,#12417,#12418));
#5946=EDGE_LOOP('',(#12419,#12420,#12421));
#5947=EDGE_LOOP('',(#12422,#12423,#12424,#12425));
#5948=EDGE_LOOP('',(#12426,#12427,#12428));
#5949=EDGE_LOOP('',(#12429,#12430,#12431));
#5950=EDGE_LOOP('',(#12432,#12433,#12434,#12435));
#5951=EDGE_LOOP('',(#12436,#12437,#12438));
#5952=EDGE_LOOP('',(#12439,#12440,#12441));
#5953=EDGE_LOOP('',(#12442,#12443,#12444,#12445));
#5954=EDGE_LOOP('',(#12446,#12447,#12448));
#5955=EDGE_LOOP('',(#12449,#12450,#12451));
#5956=EDGE_LOOP('',(#12452,#12453,#12454,#12455));
#5957=EDGE_LOOP('',(#12456,#12457,#12458));
#5958=EDGE_LOOP('',(#12459,#12460,#12461));
#5959=EDGE_LOOP('',(#12462,#12463,#12464,#12465));
#6997=CIRCLE('',#18352,30.);
#6998=CIRCLE('',#18353,5.);
#6999=CIRCLE('',#18354,25.);
#7000=CIRCLE('',#18356,250.);
#7001=CIRCLE('',#18357,250.);
#7002=CIRCLE('',#18358,5.);
#7003=CIRCLE('',#18359,245.);
#7004=CIRCLE('',#18361,35.);
#7005=CIRCLE('',#18363,35.);
#7006=CIRCLE('',#18365,35.);
#7007=CIRCLE('',#18367,35.);
#7008=CIRCLE('',#18369,35.);
#7009=CIRCLE('',#18370,35.);
#7010=CIRCLE('',#18371,35.);
#7011=CIRCLE('',#18373,35.);
#7012=CIRCLE('',#18375,35.);
#7013=CIRCLE('',#18377,35.);
#7014=CIRCLE('',#18379,35.);
#7015=CIRCLE('',#18382,2.5);
#7016=CIRCLE('',#18383,2.5);
#7017=CIRCLE('',#18385,2.49999999999997);
#7018=CIRCLE('',#18386,2.49999999999997);
#7019=CIRCLE('',#18388,2.5);
#7020=CIRCLE('',#18389,2.5);
#7021=CIRCLE('',#18391,2.5);
#7022=CIRCLE('',#18392,2.5);
#7023=CIRCLE('',#18394,2.49999999999997);
#7024=CIRCLE('',#18395,2.49999999999997);
#7025=CIRCLE('',#18397,2.5);
#7026=CIRCLE('',#18398,2.5);
#7027=CIRCLE('',#18400,2.5);
#7028=CIRCLE('',#18401,2.5);
#7029=CIRCLE('',#18403,2.5);
#7030=CIRCLE('',#18404,2.5);
#7031=CIRCLE('',#18406,19.);
#7032=CIRCLE('',#18408,19.);
#7033=CIRCLE('',#18410,15.);
#7034=CIRCLE('',#18412,15.);
#7035=CIRCLE('',#18414,25.);
#7036=CIRCLE('',#18416,2.5);
#7037=CIRCLE('',#18417,2.5);
#7038=CIRCLE('',#18419,2.5);
#7039=CIRCLE('',#18420,2.5);
#7040=CIRCLE('',#18422,2.5);
#7041=CIRCLE('',#18423,2.5);
#7042=CIRCLE('',#18425,2.5);
#7043=CIRCLE('',#18426,2.5);
#7044=CIRCLE('',#18428,2.5);
#7045=CIRCLE('',#18429,2.5);
#7046=CIRCLE('',#18431,2.5);
#7047=CIRCLE('',#18432,2.5);
#7048=CIRCLE('',#18434,2.5);
#7049=CIRCLE('',#18435,2.5);
#7050=CIRCLE('',#18437,2.5);
#7051=CIRCLE('',#18438,2.5);
#7052=CIRCLE('',#18440,2.50000000000001);
#7053=CIRCLE('',#18441,2.50000000000001);
#7054=CIRCLE('',#18443,2.5);
#7055=CIRCLE('',#18444,2.5);
#7056=CIRCLE('',#18446,2.5);
#7057=CIRCLE('',#18447,2.5);
#7058=CIRCLE('',#18449,2.5);
#7059=CIRCLE('',#18450,2.5);
#7060=CIRCLE('',#18452,2.5);
#7061=CIRCLE('',#18453,2.5);
#7062=CIRCLE('',#18455,2.5);
#7063=CIRCLE('',#18456,2.5);
#7064=CIRCLE('',#18458,2.5);
#7065=CIRCLE('',#18459,2.5);
#7066=CIRCLE('',#18461,250.);
#7067=CIRCLE('',#18463,275.);
#7068=CIRCLE('',#18464,275.);
#7069=CIRCLE('',#18466,240.);
#7070=CIRCLE('',#18467,240.);
#7071=CIRCLE('',#18473,5.);
#7072=CIRCLE('',#18474,5.);
#7073=CIRCLE('',#18475,5.00000000000003);
#7074=CIRCLE('',#18476,5.);
#7075=CIRCLE('',#18478,5.);
#7076=CIRCLE('',#18479,5.);
#7077=CIRCLE('',#18480,5.00000000000003);
#7078=CIRCLE('',#18481,5.);
#7079=CIRCLE('',#18491,5.);
#7080=CIRCLE('',#18492,5.);
#7081=CIRCLE('',#18493,5.);
#7082=CIRCLE('',#18494,5.00000000000003);
#7083=CIRCLE('',#18496,5.);
#7084=CIRCLE('',#18497,5.00000000000003);
#7085=CIRCLE('',#18498,5.);
#7086=CIRCLE('',#18499,5.);
#7676=VERTEX_POINT('',#24908);
#7677=VERTEX_POINT('',#24910);
#7678=VERTEX_POINT('',#24914);
#7679=VERTEX_POINT('',#24915);
#7680=VERTEX_POINT('',#24918);
#7681=VERTEX_POINT('',#24922);
#7682=VERTEX_POINT('',#24923);
#7683=VERTEX_POINT('',#24925);
#7684=VERTEX_POINT('',#24927);
#7685=VERTEX_POINT('',#24929);
#7686=VERTEX_POINT('',#24931);
#7687=VERTEX_POINT('',#24933);
#7688=VERTEX_POINT('',#24935);
#7689=VERTEX_POINT('',#24937);
#7690=VERTEX_POINT('',#24939);
#7691=VERTEX_POINT('',#24941);
#7692=VERTEX_POINT('',#24943);
#7693=VERTEX_POINT('',#24945);
#7694=VERTEX_POINT('',#24947);
#7695=VERTEX_POINT('',#24949);
#7696=VERTEX_POINT('',#24951);
#7697=VERTEX_POINT('',#24953);
#7698=VERTEX_POINT('',#24955);
#7699=VERTEX_POINT('',#24957);
#7700=VERTEX_POINT('',#24960);
#7701=VERTEX_POINT('',#24962);
#7702=VERTEX_POINT('',#24964);
#7703=VERTEX_POINT('',#24966);
#7704=VERTEX_POINT('',#24968);
#7705=VERTEX_POINT('',#24970);
#7706=VERTEX_POINT('',#24972);
#7707=VERTEX_POINT('',#24974);
#7708=VERTEX_POINT('',#24976);
#7709=VERTEX_POINT('',#24978);
#7710=VERTEX_POINT('',#24980);
#7711=VERTEX_POINT('',#24982);
#7712=VERTEX_POINT('',#24984);
#7713=VERTEX_POINT('',#24986);
#7714=VERTEX_POINT('',#24988);
#7715=VERTEX_POINT('',#24990);
#7716=VERTEX_POINT('',#24992);
#7717=VERTEX_POINT('',#24994);
#7718=VERTEX_POINT('',#24996);
#7719=VERTEX_POINT('',#25000);
#7720=VERTEX_POINT('',#25002);
#7721=VERTEX_POINT('',#25006);
#7722=VERTEX_POINT('',#25008);
#7723=VERTEX_POINT('',#25012);
#7724=VERTEX_POINT('',#25014);
#7725=VERTEX_POINT('',#25018);
#7726=VERTEX_POINT('',#25020);
#7727=VERTEX_POINT('',#25024);
#7728=VERTEX_POINT('',#25026);
#7729=VERTEX_POINT('',#25030);
#7730=VERTEX_POINT('',#25032);
#7731=VERTEX_POINT('',#25036);
#7732=VERTEX_POINT('',#25038);
#7733=VERTEX_POINT('',#25042);
#7734=VERTEX_POINT('',#25044);
#7735=VERTEX_POINT('',#25048);
#7736=VERTEX_POINT('',#25111);
#7737=VERTEX_POINT('',#25115);
#7738=VERTEX_POINT('',#25178);
#7739=VERTEX_POINT('',#25182);
#7740=VERTEX_POINT('',#25249);
#7741=VERTEX_POINT('',#25253);
#7742=VERTEX_POINT('',#25320);
#7743=VERTEX_POINT('',#25324);
#7744=VERTEX_POINT('',#25328);
#7745=VERTEX_POINT('',#25330);
#7746=VERTEX_POINT('',#25334);
#7747=VERTEX_POINT('',#25336);
#7748=VERTEX_POINT('',#25340);
#7749=VERTEX_POINT('',#25342);
#7750=VERTEX_POINT('',#25346);
#7751=VERTEX_POINT('',#25348);
#7752=VERTEX_POINT('',#25352);
#7753=VERTEX_POINT('',#25354);
#7754=VERTEX_POINT('',#25358);
#7755=VERTEX_POINT('',#25360);
#7756=VERTEX_POINT('',#25364);
#7757=VERTEX_POINT('',#25366);
#7758=VERTEX_POINT('',#25370);
#7759=VERTEX_POINT('',#25372);
#7760=VERTEX_POINT('',#25376);
#7761=VERTEX_POINT('',#25378);
#7762=VERTEX_POINT('',#25382);
#7763=VERTEX_POINT('',#25384);
#7764=VERTEX_POINT('',#25388);
#7765=VERTEX_POINT('',#25390);
#7766=VERTEX_POINT('',#25394);
#7767=VERTEX_POINT('',#25396);
#7768=VERTEX_POINT('',#25400);
#7769=VERTEX_POINT('',#25402);
#7770=VERTEX_POINT('',#25406);
#7771=VERTEX_POINT('',#25408);
#7772=VERTEX_POINT('',#25412);
#7773=VERTEX_POINT('',#25414);
#7774=VERTEX_POINT('',#25418);
#7775=VERTEX_POINT('',#25422);
#7776=VERTEX_POINT('',#25424);
#7777=VERTEX_POINT('',#25428);
#7778=VERTEX_POINT('',#25430);
#7779=VERTEX_POINT('',#25434);
#7780=VERTEX_POINT('',#25436);
#7781=VERTEX_POINT('',#25438);
#7782=VERTEX_POINT('',#25441);
#7783=VERTEX_POINT('',#25443);
#7784=VERTEX_POINT('',#25446);
#7785=VERTEX_POINT('',#25448);
#7786=VERTEX_POINT('',#25451);
#7787=VERTEX_POINT('',#25453);
#7788=VERTEX_POINT('',#25456);
#7789=VERTEX_POINT('',#25458);
#7790=VERTEX_POINT('',#25461);
#7791=VERTEX_POINT('',#25463);
#7792=VERTEX_POINT('',#25466);
#7793=VERTEX_POINT('',#25468);
#7794=VERTEX_POINT('',#25471);
#7795=VERTEX_POINT('',#25473);
#7796=VERTEX_POINT('',#25476);
#7797=VERTEX_POINT('',#25483);
#7798=VERTEX_POINT('',#25484);
#7799=VERTEX_POINT('',#25486);
#7800=VERTEX_POINT('',#25488);
#7801=VERTEX_POINT('',#25490);
#7802=VERTEX_POINT('',#25492);
#7803=VERTEX_POINT('',#25494);
#7804=VERTEX_POINT('',#25496);
#7805=VERTEX_POINT('',#25500);
#7806=VERTEX_POINT('',#25501);
#7807=VERTEX_POINT('',#25503);
#7808=VERTEX_POINT('',#25505);
#7809=VERTEX_POINT('',#25507);
#7810=VERTEX_POINT('',#25509);
#7811=VERTEX_POINT('',#25511);
#7812=VERTEX_POINT('',#25513);
#7813=VERTEX_POINT('',#25533);
#7814=VERTEX_POINT('',#25534);
#7815=VERTEX_POINT('',#25536);
#7816=VERTEX_POINT('',#25538);
#7817=VERTEX_POINT('',#25540);
#7818=VERTEX_POINT('',#25542);
#7819=VERTEX_POINT('',#25544);
#7820=VERTEX_POINT('',#25546);
#7821=VERTEX_POINT('',#25550);
#7822=VERTEX_POINT('',#25551);
#7823=VERTEX_POINT('',#25553);
#7824=VERTEX_POINT('',#25555);
#7825=VERTEX_POINT('',#25557);
#7826=VERTEX_POINT('',#25559);
#7827=VERTEX_POINT('',#25561);
#7828=VERTEX_POINT('',#25563);
#9383=EDGE_CURVE('',#7676,#7676,#6997,.T.);
#9384=EDGE_CURVE('',#7676,#7677,#6998,.T.);
#9385=EDGE_CURVE('',#7677,#7677,#6999,.T.);
#9386=EDGE_CURVE('',#7678,#7679,#7000,.T.);
#9387=EDGE_CURVE('',#7679,#7678,#7001,.T.);
#9388=EDGE_CURVE('',#7679,#7680,#7002,.T.);
#9389=EDGE_CURVE('',#7680,#7680,#7003,.T.);
#9390=EDGE_CURVE('',#7681,#7682,#7004,.T.);
#9391=EDGE_CURVE('',#7682,#7683,#1408,.T.);
#9392=EDGE_CURVE('',#7684,#7683,#1368,.T.);
#9393=EDGE_CURVE('',#7685,#7684,#1409,.T.);
#9394=EDGE_CURVE('',#7685,#7686,#7005,.T.);
#9395=EDGE_CURVE('',#7686,#7687,#1410,.T.);
#9396=EDGE_CURVE('',#7688,#7687,#1369,.T.);
#9397=EDGE_CURVE('',#7689,#7688,#1411,.T.);
#9398=EDGE_CURVE('',#7689,#7690,#7006,.T.);
#9399=EDGE_CURVE('',#7690,#7691,#1412,.T.);
#9400=EDGE_CURVE('',#7692,#7691,#1370,.T.);
#9401=EDGE_CURVE('',#7693,#7692,#1413,.T.);
#9402=EDGE_CURVE('',#7693,#7694,#7007,.T.);
#9403=EDGE_CURVE('',#7694,#7695,#1414,.T.);
#9404=EDGE_CURVE('',#7696,#7695,#1371,.T.);
#9405=EDGE_CURVE('',#7697,#7696,#1415,.T.);
#9406=EDGE_CURVE('',#7697,#7698,#7008,.T.);
#9407=EDGE_CURVE('',#7698,#7699,#1416,.T.);
#9408=EDGE_CURVE('',#7699,#7699,#7009,.T.);
#9409=EDGE_CURVE('',#7698,#7700,#7010,.T.);
#9410=EDGE_CURVE('',#7700,#7701,#1417,.T.);
#9411=EDGE_CURVE('',#7702,#7701,#1372,.T.);
#9412=EDGE_CURVE('',#7703,#7702,#1418,.T.);
#9413=EDGE_CURVE('',#7703,#7704,#7011,.T.);
#9414=EDGE_CURVE('',#7704,#7705,#1419,.T.);
#9415=EDGE_CURVE('',#7706,#7705,#1373,.T.);
#9416=EDGE_CURVE('',#7707,#7706,#1420,.T.);
#9417=EDGE_CURVE('',#7707,#7708,#7012,.T.);
#9418=EDGE_CURVE('',#7708,#7709,#1421,.T.);
#9419=EDGE_CURVE('',#7710,#7709,#1374,.T.);
#9420=EDGE_CURVE('',#7711,#7710,#1422,.T.);
#9421=EDGE_CURVE('',#7711,#7712,#7013,.T.);
#9422=EDGE_CURVE('',#7712,#7713,#1423,.T.);
#9423=EDGE_CURVE('',#7714,#7713,#1375,.T.);
#9424=EDGE_CURVE('',#7715,#7714,#1424,.T.);
#9425=EDGE_CURVE('',#7715,#7716,#7014,.T.);
#9426=EDGE_CURVE('',#7716,#7717,#1425,.T.);
#9427=EDGE_CURVE('',#7718,#7717,#1376,.T.);
#9428=EDGE_CURVE('',#7681,#7718,#1426,.T.);
#9429=EDGE_CURVE('',#7719,#7719,#7015,.T.);
#9430=EDGE_CURVE('',#7719,#7720,#1427,.T.);
#9431=EDGE_CURVE('',#7720,#7720,#7016,.T.);
#9432=EDGE_CURVE('',#7721,#7721,#7017,.T.);
#9433=EDGE_CURVE('',#7721,#7722,#1428,.T.);
#9434=EDGE_CURVE('',#7722,#7722,#7018,.T.);
#9435=EDGE_CURVE('',#7723,#7723,#7019,.T.);
#9436=EDGE_CURVE('',#7723,#7724,#1429,.T.);
#9437=EDGE_CURVE('',#7724,#7724,#7020,.T.);
#9438=EDGE_CURVE('',#7725,#7725,#7021,.T.);
#9439=EDGE_CURVE('',#7725,#7726,#1430,.T.);
#9440=EDGE_CURVE('',#7726,#7726,#7022,.T.);
#9441=EDGE_CURVE('',#7727,#7727,#7023,.T.);
#9442=EDGE_CURVE('',#7727,#7728,#1431,.T.);
#9443=EDGE_CURVE('',#7728,#7728,#7024,.T.);
#9444=EDGE_CURVE('',#7729,#7729,#7025,.T.);
#9445=EDGE_CURVE('',#7729,#7730,#1432,.T.);
#9446=EDGE_CURVE('',#7730,#7730,#7026,.T.);
#9447=EDGE_CURVE('',#7731,#7731,#7027,.T.);
#9448=EDGE_CURVE('',#7731,#7732,#1433,.T.);
#9449=EDGE_CURVE('',#7732,#7732,#7028,.T.);
#9450=EDGE_CURVE('',#7733,#7733,#7029,.T.);
#9451=EDGE_CURVE('',#7733,#7734,#1434,.T.);
#9452=EDGE_CURVE('',#7734,#7734,#7030,.T.);
#9453=EDGE_CURVE('',#7735,#7735,#1065,.T.);
#9454=EDGE_CURVE('',#7735,#7736,#1435,.T.);
#9455=EDGE_CURVE('',#7736,#7736,#7031,.T.);
#9456=EDGE_CURVE('',#7737,#7737,#1066,.T.);
#9457=EDGE_CURVE('',#7737,#7738,#1436,.T.);
#9458=EDGE_CURVE('',#7738,#7738,#7032,.T.);
#9459=EDGE_CURVE('',#7739,#7739,#1067,.T.);
#9460=EDGE_CURVE('',#7739,#7740,#1437,.T.);
#9461=EDGE_CURVE('',#7740,#7740,#7033,.T.);
#9462=EDGE_CURVE('',#7741,#7741,#1068,.T.);
#9463=EDGE_CURVE('',#7741,#7742,#1438,.T.);
#9464=EDGE_CURVE('',#7742,#7742,#7034,.T.);
#9465=EDGE_CURVE('',#7677,#7743,#1439,.T.);
#9466=EDGE_CURVE('',#7743,#7743,#7035,.T.);
#9467=EDGE_CURVE('',#7744,#7744,#7036,.T.);
#9468=EDGE_CURVE('',#7744,#7745,#1440,.T.);
#9469=EDGE_CURVE('',#7745,#7745,#7037,.T.);
#9470=EDGE_CURVE('',#7746,#7746,#7038,.T.);
#9471=EDGE_CURVE('',#7746,#7747,#1441,.T.);
#9472=EDGE_CURVE('',#7747,#7747,#7039,.T.);
#9473=EDGE_CURVE('',#7748,#7748,#7040,.T.);
#9474=EDGE_CURVE('',#7748,#7749,#1442,.T.);
#9475=EDGE_CURVE('',#7749,#7749,#7041,.T.);
#9476=EDGE_CURVE('',#7750,#7750,#7042,.T.);
#9477=EDGE_CURVE('',#7750,#7751,#1443,.T.);
#9478=EDGE_CURVE('',#7751,#7751,#7043,.T.);
#9479=EDGE_CURVE('',#7752,#7752,#7044,.T.);
#9480=EDGE_CURVE('',#7752,#7753,#1444,.T.);
#9481=EDGE_CURVE('',#7753,#7753,#7045,.T.);
#9482=EDGE_CURVE('',#7754,#7754,#7046,.T.);
#9483=EDGE_CURVE('',#7754,#7755,#1445,.T.);
#9484=EDGE_CURVE('',#7755,#7755,#7047,.T.);
#9485=EDGE_CURVE('',#7756,#7756,#7048,.T.);
#9486=EDGE_CURVE('',#7756,#7757,#1446,.T.);
#9487=EDGE_CURVE('',#7757,#7757,#7049,.T.);
#9488=EDGE_CURVE('',#7758,#7758,#7050,.T.);
#9489=EDGE_CURVE('',#7758,#7759,#1447,.T.);
#9490=EDGE_CURVE('',#7759,#7759,#7051,.T.);
#9491=EDGE_CURVE('',#7760,#7760,#7052,.T.);
#9492=EDGE_CURVE('',#7760,#7761,#1448,.T.);
#9493=EDGE_CURVE('',#7761,#7761,#7053,.T.);
#9494=EDGE_CURVE('',#7762,#7762,#7054,.T.);
#9495=EDGE_CURVE('',#7762,#7763,#1449,.T.);
#9496=EDGE_CURVE('',#7763,#7763,#7055,.T.);
#9497=EDGE_CURVE('',#7764,#7764,#7056,.T.);
#9498=EDGE_CURVE('',#7764,#7765,#1450,.T.);
#9499=EDGE_CURVE('',#7765,#7765,#7057,.T.);
#9500=EDGE_CURVE('',#7766,#7766,#7058,.T.);
#9501=EDGE_CURVE('',#7766,#7767,#1451,.T.);
#9502=EDGE_CURVE('',#7767,#7767,#7059,.T.);
#9503=EDGE_CURVE('',#7768,#7768,#7060,.T.);
#9504=EDGE_CURVE('',#7768,#7769,#1452,.T.);
#9505=EDGE_CURVE('',#7769,#7769,#7061,.T.);
#9506=EDGE_CURVE('',#7770,#7770,#7062,.T.);
#9507=EDGE_CURVE('',#7770,#7771,#1453,.T.);
#9508=EDGE_CURVE('',#7771,#7771,#7063,.T.);
#9509=EDGE_CURVE('',#7772,#7772,#7064,.T.);
#9510=EDGE_CURVE('',#7772,#7773,#1454,.T.);
#9511=EDGE_CURVE('',#7773,#7773,#7065,.T.);
#9512=EDGE_CURVE('',#7678,#7774,#1455,.T.);
#9513=EDGE_CURVE('',#7774,#7774,#7066,.T.);
#9514=EDGE_CURVE('',#7775,#7775,#7067,.T.);
#9515=EDGE_CURVE('',#7775,#7776,#1456,.T.);
#9516=EDGE_CURVE('',#7776,#7776,#7068,.T.);
#9517=EDGE_CURVE('',#7777,#7777,#7069,.T.);
#9518=EDGE_CURVE('',#7777,#7778,#1457,.T.);
#9519=EDGE_CURVE('',#7778,#7778,#7070,.T.);
#9520=EDGE_CURVE('',#7704,#7779,#1458,.T.);
#9521=EDGE_CURVE('',#7703,#7780,#1459,.T.);
#9522=EDGE_CURVE('',#7781,#7780,#1460,.T.);
#9523=EDGE_CURVE('',#7700,#7781,#1461,.T.);
#9524=EDGE_CURVE('',#7697,#7782,#1462,.T.);
#9525=EDGE_CURVE('',#7783,#7782,#1463,.T.);
#9526=EDGE_CURVE('',#7694,#7783,#1464,.T.);
#9527=EDGE_CURVE('',#7693,#7784,#1465,.T.);
#9528=EDGE_CURVE('',#7785,#7784,#1466,.T.);
#9529=EDGE_CURVE('',#7690,#7785,#1467,.T.);
#9530=EDGE_CURVE('',#7689,#7786,#1468,.T.);
#9531=EDGE_CURVE('',#7787,#7786,#1469,.T.);
#9532=EDGE_CURVE('',#7686,#7787,#1470,.T.);
#9533=EDGE_CURVE('',#7685,#7788,#1471,.T.);
#9534=EDGE_CURVE('',#7789,#7788,#1472,.T.);
#9535=EDGE_CURVE('',#7682,#7789,#1473,.T.);
#9536=EDGE_CURVE('',#7681,#7790,#1474,.T.);
#9537=EDGE_CURVE('',#7791,#7790,#1475,.T.);
#9538=EDGE_CURVE('',#7716,#7791,#1476,.T.);
#9539=EDGE_CURVE('',#7715,#7792,#1477,.T.);
#9540=EDGE_CURVE('',#7793,#7792,#1478,.T.);
#9541=EDGE_CURVE('',#7712,#7793,#1479,.T.);
#9542=EDGE_CURVE('',#7711,#7794,#1480,.T.);
#9543=EDGE_CURVE('',#7795,#7794,#1481,.T.);
#9544=EDGE_CURVE('',#7708,#7795,#1482,.T.);
#9545=EDGE_CURVE('',#7707,#7796,#1483,.T.);
#9546=EDGE_CURVE('',#7779,#7796,#1484,.T.);
#9547=EDGE_CURVE('',#7797,#7798,#7071,.T.);
#9548=EDGE_CURVE('',#7798,#7799,#1485,.T.);
#9549=EDGE_CURVE('',#7799,#7800,#7072,.T.);
#9550=EDGE_CURVE('',#7800,#7801,#1486,.T.);
#9551=EDGE_CURVE('',#7801,#7802,#7073,.T.);
#9552=EDGE_CURVE('',#7802,#7803,#1487,.T.);
#9553=EDGE_CURVE('',#7803,#7804,#7074,.T.);
#9554=EDGE_CURVE('',#7804,#7797,#1488,.T.);
#9555=EDGE_CURVE('',#7805,#7806,#7075,.T.);
#9556=EDGE_CURVE('',#7807,#7805,#1489,.T.);
#9557=EDGE_CURVE('',#7808,#7807,#7076,.T.);
#9558=EDGE_CURVE('',#7809,#7808,#1490,.T.);
#9559=EDGE_CURVE('',#7810,#7809,#7077,.T.);
#9560=EDGE_CURVE('',#7811,#7810,#1491,.T.);
#9561=EDGE_CURVE('',#7812,#7811,#7078,.T.);
#9562=EDGE_CURVE('',#7806,#7812,#1492,.T.);
#9563=EDGE_CURVE('',#7798,#7806,#1493,.T.);
#9564=EDGE_CURVE('',#7797,#7805,#1494,.T.);
#9565=EDGE_CURVE('',#7799,#7812,#1495,.T.);
#9566=EDGE_CURVE('',#7800,#7811,#1496,.T.);
#9567=EDGE_CURVE('',#7801,#7810,#1497,.T.);
#9568=EDGE_CURVE('',#7802,#7809,#1498,.T.);
#9569=EDGE_CURVE('',#7803,#7808,#1499,.T.);
#9570=EDGE_CURVE('',#7804,#7807,#1500,.T.);
#9571=EDGE_CURVE('',#7813,#7814,#7079,.T.);
#9572=EDGE_CURVE('',#7814,#7815,#1501,.T.);
#9573=EDGE_CURVE('',#7815,#7816,#7080,.T.);
#9574=EDGE_CURVE('',#7816,#7817,#1502,.T.);
#9575=EDGE_CURVE('',#7817,#7818,#7081,.T.);
#9576=EDGE_CURVE('',#7818,#7819,#1503,.T.);
#9577=EDGE_CURVE('',#7819,#7820,#7082,.T.);
#9578=EDGE_CURVE('',#7820,#7813,#1504,.T.);
#9579=EDGE_CURVE('',#7821,#7822,#7083,.T.);
#9580=EDGE_CURVE('',#7823,#7821,#1505,.T.);
#9581=EDGE_CURVE('',#7824,#7823,#7084,.T.);
#9582=EDGE_CURVE('',#7825,#7824,#1506,.T.);
#9583=EDGE_CURVE('',#7826,#7825,#7085,.T.);
#9584=EDGE_CURVE('',#7827,#7826,#1507,.T.);
#9585=EDGE_CURVE('',#7828,#7827,#7086,.T.);
#9586=EDGE_CURVE('',#7822,#7828,#1508,.T.);
#9587=EDGE_CURVE('',#7814,#7822,#1509,.T.);
#9588=EDGE_CURVE('',#7813,#7821,#1510,.T.);
#9589=EDGE_CURVE('',#7815,#7828,#1511,.T.);
#9590=EDGE_CURVE('',#7816,#7827,#1512,.T.);
#9591=EDGE_CURVE('',#7817,#7826,#1513,.T.);
#9592=EDGE_CURVE('',#7818,#7825,#1514,.T.);
#9593=EDGE_CURVE('',#7819,#7824,#1515,.T.);
#9594=EDGE_CURVE('',#7820,#7823,#1516,.T.);
#9595=EDGE_CURVE('',#7795,#7709,#1517,.T.);
#9596=EDGE_CURVE('',#7794,#7710,#1518,.T.);
#9597=EDGE_CURVE('',#7793,#7713,#1519,.T.);
#9598=EDGE_CURVE('',#7792,#7714,#1520,.T.);
#9599=EDGE_CURVE('',#7791,#7717,#1521,.T.);
#9600=EDGE_CURVE('',#7790,#7718,#1522,.T.);
#9601=EDGE_CURVE('',#7789,#7683,#1523,.T.);
#9602=EDGE_CURVE('',#7788,#7684,#1524,.T.);
#9603=EDGE_CURVE('',#7787,#7687,#1525,.T.);
#9604=EDGE_CURVE('',#7786,#7688,#1526,.T.);
#9605=EDGE_CURVE('',#7785,#7691,#1527,.T.);
#9606=EDGE_CURVE('',#7784,#7692,#1528,.T.);
#9607=EDGE_CURVE('',#7783,#7695,#1529,.T.);
#9608=EDGE_CURVE('',#7782,#7696,#1530,.T.);
#9609=EDGE_CURVE('',#7781,#7701,#1531,.T.);
#9610=EDGE_CURVE('',#7780,#7702,#1532,.T.);
#9611=EDGE_CURVE('',#7779,#7705,#1533,.T.);
#9612=EDGE_CURVE('',#7796,#7706,#1534,.T.);
#12006=ORIENTED_EDGE('',*,*,#9383,.F.);
#12007=ORIENTED_EDGE('',*,*,#9384,.T.);
#12008=ORIENTED_EDGE('',*,*,#9385,.F.);
#12009=ORIENTED_EDGE('',*,*,#9384,.F.);
#12010=ORIENTED_EDGE('',*,*,#9386,.F.);
#12011=ORIENTED_EDGE('',*,*,#9387,.F.);
#12012=ORIENTED_EDGE('',*,*,#9388,.T.);
#12013=ORIENTED_EDGE('',*,*,#9389,.F.);
#12014=ORIENTED_EDGE('',*,*,#9388,.F.);
#12015=ORIENTED_EDGE('',*,*,#9390,.T.);
#12016=ORIENTED_EDGE('',*,*,#9391,.T.);
#12017=ORIENTED_EDGE('',*,*,#9392,.F.);
#12018=ORIENTED_EDGE('',*,*,#9393,.F.);
#12019=ORIENTED_EDGE('',*,*,#9394,.T.);
#12020=ORIENTED_EDGE('',*,*,#9395,.T.);
#12021=ORIENTED_EDGE('',*,*,#9396,.F.);
#12022=ORIENTED_EDGE('',*,*,#9397,.F.);
#12023=ORIENTED_EDGE('',*,*,#9398,.T.);
#12024=ORIENTED_EDGE('',*,*,#9399,.T.);
#12025=ORIENTED_EDGE('',*,*,#9400,.F.);
#12026=ORIENTED_EDGE('',*,*,#9401,.F.);
#12027=ORIENTED_EDGE('',*,*,#9402,.T.);
#12028=ORIENTED_EDGE('',*,*,#9403,.T.);
#12029=ORIENTED_EDGE('',*,*,#9404,.F.);
#12030=ORIENTED_EDGE('',*,*,#9405,.F.);
#12031=ORIENTED_EDGE('',*,*,#9406,.T.);
#12032=ORIENTED_EDGE('',*,*,#9407,.T.);
#12033=ORIENTED_EDGE('',*,*,#9408,.F.);
#12034=ORIENTED_EDGE('',*,*,#9407,.F.);
#12035=ORIENTED_EDGE('',*,*,#9409,.T.);
#12036=ORIENTED_EDGE('',*,*,#9410,.T.);
#12037=ORIENTED_EDGE('',*,*,#9411,.F.);
#12038=ORIENTED_EDGE('',*,*,#9412,.F.);
#12039=ORIENTED_EDGE('',*,*,#9413,.T.);
#12040=ORIENTED_EDGE('',*,*,#9414,.T.);
#12041=ORIENTED_EDGE('',*,*,#9415,.F.);
#12042=ORIENTED_EDGE('',*,*,#9416,.F.);
#12043=ORIENTED_EDGE('',*,*,#9417,.T.);
#12044=ORIENTED_EDGE('',*,*,#9418,.T.);
#12045=ORIENTED_EDGE('',*,*,#9419,.F.);
#12046=ORIENTED_EDGE('',*,*,#9420,.F.);
#12047=ORIENTED_EDGE('',*,*,#9421,.T.);
#12048=ORIENTED_EDGE('',*,*,#9422,.T.);
#12049=ORIENTED_EDGE('',*,*,#9423,.F.);
#12050=ORIENTED_EDGE('',*,*,#9424,.F.);
#12051=ORIENTED_EDGE('',*,*,#9425,.T.);
#12052=ORIENTED_EDGE('',*,*,#9426,.T.);
#12053=ORIENTED_EDGE('',*,*,#9427,.F.);
#12054=ORIENTED_EDGE('',*,*,#9428,.F.);
#12055=ORIENTED_EDGE('',*,*,#9429,.T.);
#12056=ORIENTED_EDGE('',*,*,#9430,.T.);
#12057=ORIENTED_EDGE('',*,*,#9431,.F.);
#12058=ORIENTED_EDGE('',*,*,#9430,.F.);
#12059=ORIENTED_EDGE('',*,*,#9432,.T.);
#12060=ORIENTED_EDGE('',*,*,#9433,.T.);
#12061=ORIENTED_EDGE('',*,*,#9434,.F.);
#12062=ORIENTED_EDGE('',*,*,#9433,.F.);
#12063=ORIENTED_EDGE('',*,*,#9435,.T.);
#12064=ORIENTED_EDGE('',*,*,#9436,.T.);
#12065=ORIENTED_EDGE('',*,*,#9437,.F.);
#12066=ORIENTED_EDGE('',*,*,#9436,.F.);
#12067=ORIENTED_EDGE('',*,*,#9438,.T.);
#12068=ORIENTED_EDGE('',*,*,#9439,.T.);
#12069=ORIENTED_EDGE('',*,*,#9440,.F.);
#12070=ORIENTED_EDGE('',*,*,#9439,.F.);
#12071=ORIENTED_EDGE('',*,*,#9441,.T.);
#12072=ORIENTED_EDGE('',*,*,#9442,.T.);
#12073=ORIENTED_EDGE('',*,*,#9443,.F.);
#12074=ORIENTED_EDGE('',*,*,#9442,.F.);
#12075=ORIENTED_EDGE('',*,*,#9444,.T.);
#12076=ORIENTED_EDGE('',*,*,#9445,.T.);
#12077=ORIENTED_EDGE('',*,*,#9446,.F.);
#12078=ORIENTED_EDGE('',*,*,#9445,.F.);
#12079=ORIENTED_EDGE('',*,*,#9447,.T.);
#12080=ORIENTED_EDGE('',*,*,#9448,.T.);
#12081=ORIENTED_EDGE('',*,*,#9449,.F.);
#12082=ORIENTED_EDGE('',*,*,#9448,.F.);
#12083=ORIENTED_EDGE('',*,*,#9450,.T.);
#12084=ORIENTED_EDGE('',*,*,#9451,.T.);
#12085=ORIENTED_EDGE('',*,*,#9452,.F.);
#12086=ORIENTED_EDGE('',*,*,#9451,.F.);
#12087=ORIENTED_EDGE('',*,*,#9453,.F.);
#12088=ORIENTED_EDGE('',*,*,#9454,.T.);
#12089=ORIENTED_EDGE('',*,*,#9455,.T.);
#12090=ORIENTED_EDGE('',*,*,#9454,.F.);
#12091=ORIENTED_EDGE('',*,*,#9456,.F.);
#12092=ORIENTED_EDGE('',*,*,#9457,.T.);
#12093=ORIENTED_EDGE('',*,*,#9458,.T.);
#12094=ORIENTED_EDGE('',*,*,#9457,.F.);
#12095=ORIENTED_EDGE('',*,*,#9459,.F.);
#12096=ORIENTED_EDGE('',*,*,#9460,.T.);
#12097=ORIENTED_EDGE('',*,*,#9461,.T.);
#12098=ORIENTED_EDGE('',*,*,#9460,.F.);
#12099=ORIENTED_EDGE('',*,*,#9462,.F.);
#12100=ORIENTED_EDGE('',*,*,#9463,.T.);
#12101=ORIENTED_EDGE('',*,*,#9464,.T.);
#12102=ORIENTED_EDGE('',*,*,#9463,.F.);
#12103=ORIENTED_EDGE('',*,*,#9385,.T.);
#12104=ORIENTED_EDGE('',*,*,#9465,.T.);
#12105=ORIENTED_EDGE('',*,*,#9466,.T.);
#12106=ORIENTED_EDGE('',*,*,#9465,.F.);
#12107=ORIENTED_EDGE('',*,*,#9467,.F.);
#12108=ORIENTED_EDGE('',*,*,#9468,.T.);
#12109=ORIENTED_EDGE('',*,*,#9469,.T.);
#12110=ORIENTED_EDGE('',*,*,#9468,.F.);
#12111=ORIENTED_EDGE('',*,*,#9470,.F.);
#12112=ORIENTED_EDGE('',*,*,#9471,.T.);
#12113=ORIENTED_EDGE('',*,*,#9472,.T.);
#12114=ORIENTED_EDGE('',*,*,#9471,.F.);
#12115=ORIENTED_EDGE('',*,*,#9473,.F.);
#12116=ORIENTED_EDGE('',*,*,#9474,.T.);
#12117=ORIENTED_EDGE('',*,*,#9475,.T.);
#12118=ORIENTED_EDGE('',*,*,#9474,.F.);
#12119=ORIENTED_EDGE('',*,*,#9476,.F.);
#12120=ORIENTED_EDGE('',*,*,#9477,.T.);
#12121=ORIENTED_EDGE('',*,*,#9478,.T.);
#12122=ORIENTED_EDGE('',*,*,#9477,.F.);
#12123=ORIENTED_EDGE('',*,*,#9479,.F.);
#12124=ORIENTED_EDGE('',*,*,#9480,.T.);
#12125=ORIENTED_EDGE('',*,*,#9481,.T.);
#12126=ORIENTED_EDGE('',*,*,#9480,.F.);
#12127=ORIENTED_EDGE('',*,*,#9482,.F.);
#12128=ORIENTED_EDGE('',*,*,#9483,.T.);
#12129=ORIENTED_EDGE('',*,*,#9484,.T.);
#12130=ORIENTED_EDGE('',*,*,#9483,.F.);
#12131=ORIENTED_EDGE('',*,*,#9485,.F.);
#12132=ORIENTED_EDGE('',*,*,#9486,.T.);
#12133=ORIENTED_EDGE('',*,*,#9487,.T.);
#12134=ORIENTED_EDGE('',*,*,#9486,.F.);
#12135=ORIENTED_EDGE('',*,*,#9488,.F.);
#12136=ORIENTED_EDGE('',*,*,#9489,.T.);
#12137=ORIENTED_EDGE('',*,*,#9490,.T.);
#12138=ORIENTED_EDGE('',*,*,#9489,.F.);
#12139=ORIENTED_EDGE('',*,*,#9491,.F.);
#12140=ORIENTED_EDGE('',*,*,#9492,.T.);
#12141=ORIENTED_EDGE('',*,*,#9493,.T.);
#12142=ORIENTED_EDGE('',*,*,#9492,.F.);
#12143=ORIENTED_EDGE('',*,*,#9494,.F.);
#12144=ORIENTED_EDGE('',*,*,#9495,.T.);
#12145=ORIENTED_EDGE('',*,*,#9496,.T.);
#12146=ORIENTED_EDGE('',*,*,#9495,.F.);
#12147=ORIENTED_EDGE('',*,*,#9497,.F.);
#12148=ORIENTED_EDGE('',*,*,#9498,.T.);
#12149=ORIENTED_EDGE('',*,*,#9499,.T.);
#12150=ORIENTED_EDGE('',*,*,#9498,.F.);
#12151=ORIENTED_EDGE('',*,*,#9500,.F.);
#12152=ORIENTED_EDGE('',*,*,#9501,.T.);
#12153=ORIENTED_EDGE('',*,*,#9502,.T.);
#12154=ORIENTED_EDGE('',*,*,#9501,.F.);
#12155=ORIENTED_EDGE('',*,*,#9503,.F.);
#12156=ORIENTED_EDGE('',*,*,#9504,.T.);
#12157=ORIENTED_EDGE('',*,*,#9505,.T.);
#12158=ORIENTED_EDGE('',*,*,#9504,.F.);
#12159=ORIENTED_EDGE('',*,*,#9506,.F.);
#12160=ORIENTED_EDGE('',*,*,#9507,.T.);
#12161=ORIENTED_EDGE('',*,*,#9508,.T.);
#12162=ORIENTED_EDGE('',*,*,#9507,.F.);
#12163=ORIENTED_EDGE('',*,*,#9509,.F.);
#12164=ORIENTED_EDGE('',*,*,#9510,.T.);
#12165=ORIENTED_EDGE('',*,*,#9511,.T.);
#12166=ORIENTED_EDGE('',*,*,#9510,.F.);
#12167=ORIENTED_EDGE('',*,*,#9386,.T.);
#12168=ORIENTED_EDGE('',*,*,#9387,.T.);
#12169=ORIENTED_EDGE('',*,*,#9512,.T.);
#12170=ORIENTED_EDGE('',*,*,#9513,.F.);
#12171=ORIENTED_EDGE('',*,*,#9512,.F.);
#12172=ORIENTED_EDGE('',*,*,#9456,.T.);
#12173=ORIENTED_EDGE('',*,*,#9453,.T.);
#12174=ORIENTED_EDGE('',*,*,#9514,.F.);
#12175=ORIENTED_EDGE('',*,*,#9515,.T.);
#12176=ORIENTED_EDGE('',*,*,#9516,.T.);
#12177=ORIENTED_EDGE('',*,*,#9515,.F.);
#12178=ORIENTED_EDGE('',*,*,#9517,.T.);
#12179=ORIENTED_EDGE('',*,*,#9518,.T.);
#12180=ORIENTED_EDGE('',*,*,#9519,.T.);
#12181=ORIENTED_EDGE('',*,*,#9518,.F.);
#12182=ORIENTED_EDGE('',*,*,#9462,.T.);
#12183=ORIENTED_EDGE('',*,*,#9459,.T.);
#12184=ORIENTED_EDGE('',*,*,#9517,.F.);
#12185=ORIENTED_EDGE('',*,*,#9520,.F.);
#12186=ORIENTED_EDGE('',*,*,#9413,.F.);
#12187=ORIENTED_EDGE('',*,*,#9521,.T.);
#12188=ORIENTED_EDGE('',*,*,#9522,.F.);
#12189=ORIENTED_EDGE('',*,*,#9523,.F.);
#12190=ORIENTED_EDGE('',*,*,#9409,.F.);
#12191=ORIENTED_EDGE('',*,*,#9406,.F.);
#12192=ORIENTED_EDGE('',*,*,#9524,.T.);
#12193=ORIENTED_EDGE('',*,*,#9525,.F.);
#12194=ORIENTED_EDGE('',*,*,#9526,.F.);
#12195=ORIENTED_EDGE('',*,*,#9402,.F.);
#12196=ORIENTED_EDGE('',*,*,#9527,.T.);
#12197=ORIENTED_EDGE('',*,*,#9528,.F.);
#12198=ORIENTED_EDGE('',*,*,#9529,.F.);
#12199=ORIENTED_EDGE('',*,*,#9398,.F.);
#12200=ORIENTED_EDGE('',*,*,#9530,.T.);
#12201=ORIENTED_EDGE('',*,*,#9531,.F.);
#12202=ORIENTED_EDGE('',*,*,#9532,.F.);
#12203=ORIENTED_EDGE('',*,*,#9394,.F.);
#12204=ORIENTED_EDGE('',*,*,#9533,.T.);
#12205=ORIENTED_EDGE('',*,*,#9534,.F.);
#12206=ORIENTED_EDGE('',*,*,#9535,.F.);
#12207=ORIENTED_EDGE('',*,*,#9390,.F.);
#12208=ORIENTED_EDGE('',*,*,#9536,.T.);
#12209=ORIENTED_EDGE('',*,*,#9537,.F.);
#12210=ORIENTED_EDGE('',*,*,#9538,.F.);
#12211=ORIENTED_EDGE('',*,*,#9425,.F.);
#12212=ORIENTED_EDGE('',*,*,#9539,.T.);
#12213=ORIENTED_EDGE('',*,*,#9540,.F.);
#12214=ORIENTED_EDGE('',*,*,#9541,.F.);
#12215=ORIENTED_EDGE('',*,*,#9421,.F.);
#12216=ORIENTED_EDGE('',*,*,#9542,.T.);
#12217=ORIENTED_EDGE('',*,*,#9543,.F.);
#12218=ORIENTED_EDGE('',*,*,#9544,.F.);
#12219=ORIENTED_EDGE('',*,*,#9417,.F.);
#12220=ORIENTED_EDGE('',*,*,#9545,.T.);
#12221=ORIENTED_EDGE('',*,*,#9546,.F.);
#12222=ORIENTED_EDGE('',*,*,#9514,.T.);
#12223=ORIENTED_EDGE('',*,*,#9469,.F.);
#12224=ORIENTED_EDGE('',*,*,#9472,.F.);
#12225=ORIENTED_EDGE('',*,*,#9475,.F.);
#12226=ORIENTED_EDGE('',*,*,#9478,.F.);
#12227=ORIENTED_EDGE('',*,*,#9481,.F.);
#12228=ORIENTED_EDGE('',*,*,#9484,.F.);
#12229=ORIENTED_EDGE('',*,*,#9487,.F.);
#12230=ORIENTED_EDGE('',*,*,#9490,.F.);
#12231=ORIENTED_EDGE('',*,*,#9493,.F.);
#12232=ORIENTED_EDGE('',*,*,#9496,.F.);
#12233=ORIENTED_EDGE('',*,*,#9499,.F.);
#12234=ORIENTED_EDGE('',*,*,#9502,.F.);
#12235=ORIENTED_EDGE('',*,*,#9505,.F.);
#12236=ORIENTED_EDGE('',*,*,#9508,.F.);
#12237=ORIENTED_EDGE('',*,*,#9511,.F.);
#12238=ORIENTED_EDGE('',*,*,#9519,.F.);
#12239=ORIENTED_EDGE('',*,*,#9516,.F.);
#12240=ORIENTED_EDGE('',*,*,#9513,.T.);
#12241=ORIENTED_EDGE('',*,*,#9467,.T.);
#12242=ORIENTED_EDGE('',*,*,#9470,.T.);
#12243=ORIENTED_EDGE('',*,*,#9473,.T.);
#12244=ORIENTED_EDGE('',*,*,#9476,.T.);
#12245=ORIENTED_EDGE('',*,*,#9479,.T.);
#12246=ORIENTED_EDGE('',*,*,#9482,.T.);
#12247=ORIENTED_EDGE('',*,*,#9485,.T.);
#12248=ORIENTED_EDGE('',*,*,#9488,.T.);
#12249=ORIENTED_EDGE('',*,*,#9491,.T.);
#12250=ORIENTED_EDGE('',*,*,#9494,.T.);
#12251=ORIENTED_EDGE('',*,*,#9497,.T.);
#12252=ORIENTED_EDGE('',*,*,#9500,.T.);
#12253=ORIENTED_EDGE('',*,*,#9503,.T.);
#12254=ORIENTED_EDGE('',*,*,#9506,.T.);
#12255=ORIENTED_EDGE('',*,*,#9509,.T.);
#12256=ORIENTED_EDGE('',*,*,#9389,.T.);
#12257=ORIENTED_EDGE('',*,*,#9383,.T.);
#12258=ORIENTED_EDGE('',*,*,#9547,.T.);
#12259=ORIENTED_EDGE('',*,*,#9548,.T.);
#12260=ORIENTED_EDGE('',*,*,#9549,.T.);
#12261=ORIENTED_EDGE('',*,*,#9550,.T.);
#12262=ORIENTED_EDGE('',*,*,#9551,.T.);
#12263=ORIENTED_EDGE('',*,*,#9552,.T.);
#12264=ORIENTED_EDGE('',*,*,#9553,.T.);
#12265=ORIENTED_EDGE('',*,*,#9554,.T.);
#12266=ORIENTED_EDGE('',*,*,#9450,.F.);
#12267=ORIENTED_EDGE('',*,*,#9444,.F.);
#12268=ORIENTED_EDGE('',*,*,#9464,.F.);
#12269=ORIENTED_EDGE('',*,*,#9441,.F.);
#12270=ORIENTED_EDGE('',*,*,#9447,.F.);
#12271=ORIENTED_EDGE('',*,*,#9555,.F.);
#12272=ORIENTED_EDGE('',*,*,#9556,.F.);
#12273=ORIENTED_EDGE('',*,*,#9557,.F.);
#12274=ORIENTED_EDGE('',*,*,#9558,.F.);
#12275=ORIENTED_EDGE('',*,*,#9559,.F.);
#12276=ORIENTED_EDGE('',*,*,#9560,.F.);
#12277=ORIENTED_EDGE('',*,*,#9561,.F.);
#12278=ORIENTED_EDGE('',*,*,#9562,.F.);
#12279=ORIENTED_EDGE('',*,*,#9452,.T.);
#12280=ORIENTED_EDGE('',*,*,#9449,.T.);
#12281=ORIENTED_EDGE('',*,*,#9446,.T.);
#12282=ORIENTED_EDGE('',*,*,#9443,.T.);
#12283=ORIENTED_EDGE('',*,*,#9455,.F.);
#12284=ORIENTED_EDGE('',*,*,#9555,.T.);
#12285=ORIENTED_EDGE('',*,*,#9563,.F.);
#12286=ORIENTED_EDGE('',*,*,#9547,.F.);
#12287=ORIENTED_EDGE('',*,*,#9564,.T.);
#12288=ORIENTED_EDGE('',*,*,#9562,.T.);
#12289=ORIENTED_EDGE('',*,*,#9565,.F.);
#12290=ORIENTED_EDGE('',*,*,#9548,.F.);
#12291=ORIENTED_EDGE('',*,*,#9563,.T.);
#12292=ORIENTED_EDGE('',*,*,#9561,.T.);
#12293=ORIENTED_EDGE('',*,*,#9566,.F.);
#12294=ORIENTED_EDGE('',*,*,#9549,.F.);
#12295=ORIENTED_EDGE('',*,*,#9565,.T.);
#12296=ORIENTED_EDGE('',*,*,#9560,.T.);
#12297=ORIENTED_EDGE('',*,*,#9567,.F.);
#12298=ORIENTED_EDGE('',*,*,#9550,.F.);
#12299=ORIENTED_EDGE('',*,*,#9566,.T.);
#12300=ORIENTED_EDGE('',*,*,#9559,.T.);
#12301=ORIENTED_EDGE('',*,*,#9568,.F.);
#12302=ORIENTED_EDGE('',*,*,#9551,.F.);
#12303=ORIENTED_EDGE('',*,*,#9567,.T.);
#12304=ORIENTED_EDGE('',*,*,#9558,.T.);
#12305=ORIENTED_EDGE('',*,*,#9569,.F.);
#12306=ORIENTED_EDGE('',*,*,#9552,.F.);
#12307=ORIENTED_EDGE('',*,*,#9568,.T.);
#12308=ORIENTED_EDGE('',*,*,#9557,.T.);
#12309=ORIENTED_EDGE('',*,*,#9570,.F.);
#12310=ORIENTED_EDGE('',*,*,#9553,.F.);
#12311=ORIENTED_EDGE('',*,*,#9569,.T.);
#12312=ORIENTED_EDGE('',*,*,#9556,.T.);
#12313=ORIENTED_EDGE('',*,*,#9564,.F.);
#12314=ORIENTED_EDGE('',*,*,#9554,.F.);
#12315=ORIENTED_EDGE('',*,*,#9570,.T.);
#12316=ORIENTED_EDGE('',*,*,#9571,.T.);
#12317=ORIENTED_EDGE('',*,*,#9572,.T.);
#12318=ORIENTED_EDGE('',*,*,#9573,.T.);
#12319=ORIENTED_EDGE('',*,*,#9574,.T.);
#12320=ORIENTED_EDGE('',*,*,#9575,.T.);
#12321=ORIENTED_EDGE('',*,*,#9576,.T.);
#12322=ORIENTED_EDGE('',*,*,#9577,.T.);
#12323=ORIENTED_EDGE('',*,*,#9578,.T.);
#12324=ORIENTED_EDGE('',*,*,#9461,.F.);
#12325=ORIENTED_EDGE('',*,*,#9435,.F.);
#12326=ORIENTED_EDGE('',*,*,#9429,.F.);
#12327=ORIENTED_EDGE('',*,*,#9432,.F.);
#12328=ORIENTED_EDGE('',*,*,#9438,.F.);
#12329=ORIENTED_EDGE('',*,*,#9579,.F.);
#12330=ORIENTED_EDGE('',*,*,#9580,.F.);
#12331=ORIENTED_EDGE('',*,*,#9581,.F.);
#12332=ORIENTED_EDGE('',*,*,#9582,.F.);
#12333=ORIENTED_EDGE('',*,*,#9583,.F.);
#12334=ORIENTED_EDGE('',*,*,#9584,.F.);
#12335=ORIENTED_EDGE('',*,*,#9585,.F.);
#12336=ORIENTED_EDGE('',*,*,#9586,.F.);
#12337=ORIENTED_EDGE('',*,*,#9440,.T.);
#12338=ORIENTED_EDGE('',*,*,#9437,.T.);
#12339=ORIENTED_EDGE('',*,*,#9434,.T.);
#12340=ORIENTED_EDGE('',*,*,#9431,.T.);
#12341=ORIENTED_EDGE('',*,*,#9458,.F.);
#12342=ORIENTED_EDGE('',*,*,#9579,.T.);
#12343=ORIENTED_EDGE('',*,*,#9587,.F.);
#12344=ORIENTED_EDGE('',*,*,#9571,.F.);
#12345=ORIENTED_EDGE('',*,*,#9588,.T.);
#12346=ORIENTED_EDGE('',*,*,#9586,.T.);
#12347=ORIENTED_EDGE('',*,*,#9589,.F.);
#12348=ORIENTED_EDGE('',*,*,#9572,.F.);
#12349=ORIENTED_EDGE('',*,*,#9587,.T.);
#12350=ORIENTED_EDGE('',*,*,#9585,.T.);
#12351=ORIENTED_EDGE('',*,*,#9590,.F.);
#12352=ORIENTED_EDGE('',*,*,#9573,.F.);
#12353=ORIENTED_EDGE('',*,*,#9589,.T.);
#12354=ORIENTED_EDGE('',*,*,#9584,.T.);
#12355=ORIENTED_EDGE('',*,*,#9591,.F.);
#12356=ORIENTED_EDGE('',*,*,#9574,.F.);
#12357=ORIENTED_EDGE('',*,*,#9590,.T.);
#12358=ORIENTED_EDGE('',*,*,#9583,.T.);
#12359=ORIENTED_EDGE('',*,*,#9592,.F.);
#12360=ORIENTED_EDGE('',*,*,#9575,.F.);
#12361=ORIENTED_EDGE('',*,*,#9591,.T.);
#12362=ORIENTED_EDGE('',*,*,#9582,.T.);
#12363=ORIENTED_EDGE('',*,*,#9593,.F.);
#12364=ORIENTED_EDGE('',*,*,#9576,.F.);
#12365=ORIENTED_EDGE('',*,*,#9592,.T.);
#12366=ORIENTED_EDGE('',*,*,#9581,.T.);
#12367=ORIENTED_EDGE('',*,*,#9594,.F.);
#12368=ORIENTED_EDGE('',*,*,#9577,.F.);
#12369=ORIENTED_EDGE('',*,*,#9593,.T.);
#12370=ORIENTED_EDGE('',*,*,#9580,.T.);
#12371=ORIENTED_EDGE('',*,*,#9588,.F.);
#12372=ORIENTED_EDGE('',*,*,#9578,.F.);
#12373=ORIENTED_EDGE('',*,*,#9594,.T.);
#12374=ORIENTED_EDGE('',*,*,#9408,.T.);
#12375=ORIENTED_EDGE('',*,*,#9466,.F.);
#12376=ORIENTED_EDGE('',*,*,#9418,.F.);
#12377=ORIENTED_EDGE('',*,*,#9544,.T.);
#12378=ORIENTED_EDGE('',*,*,#9595,.T.);
#12379=ORIENTED_EDGE('',*,*,#9542,.F.);
#12380=ORIENTED_EDGE('',*,*,#9420,.T.);
#12381=ORIENTED_EDGE('',*,*,#9596,.F.);
#12382=ORIENTED_EDGE('',*,*,#9596,.T.);
#12383=ORIENTED_EDGE('',*,*,#9419,.T.);
#12384=ORIENTED_EDGE('',*,*,#9595,.F.);
#12385=ORIENTED_EDGE('',*,*,#9543,.T.);
#12386=ORIENTED_EDGE('',*,*,#9422,.F.);
#12387=ORIENTED_EDGE('',*,*,#9541,.T.);
#12388=ORIENTED_EDGE('',*,*,#9597,.T.);
#12389=ORIENTED_EDGE('',*,*,#9539,.F.);
#12390=ORIENTED_EDGE('',*,*,#9424,.T.);
#12391=ORIENTED_EDGE('',*,*,#9598,.F.);
#12392=ORIENTED_EDGE('',*,*,#9598,.T.);
#12393=ORIENTED_EDGE('',*,*,#9423,.T.);
#12394=ORIENTED_EDGE('',*,*,#9597,.F.);
#12395=ORIENTED_EDGE('',*,*,#9540,.T.);
#12396=ORIENTED_EDGE('',*,*,#9426,.F.);
#12397=ORIENTED_EDGE('',*,*,#9538,.T.);
#12398=ORIENTED_EDGE('',*,*,#9599,.T.);
#12399=ORIENTED_EDGE('',*,*,#9536,.F.);
#12400=ORIENTED_EDGE('',*,*,#9428,.T.);
#12401=ORIENTED_EDGE('',*,*,#9600,.F.);
#12402=ORIENTED_EDGE('',*,*,#9600,.T.);
#12403=ORIENTED_EDGE('',*,*,#9427,.T.);
#12404=ORIENTED_EDGE('',*,*,#9599,.F.);
#12405=ORIENTED_EDGE('',*,*,#9537,.T.);
#12406=ORIENTED_EDGE('',*,*,#9391,.F.);
#12407=ORIENTED_EDGE('',*,*,#9535,.T.);
#12408=ORIENTED_EDGE('',*,*,#9601,.T.);
#12409=ORIENTED_EDGE('',*,*,#9533,.F.);
#12410=ORIENTED_EDGE('',*,*,#9393,.T.);
#12411=ORIENTED_EDGE('',*,*,#9602,.F.);
#12412=ORIENTED_EDGE('',*,*,#9602,.T.);
#12413=ORIENTED_EDGE('',*,*,#9392,.T.);
#12414=ORIENTED_EDGE('',*,*,#9601,.F.);
#12415=ORIENTED_EDGE('',*,*,#9534,.T.);
#12416=ORIENTED_EDGE('',*,*,#9395,.F.);
#12417=ORIENTED_EDGE('',*,*,#9532,.T.);
#12418=ORIENTED_EDGE('',*,*,#9603,.T.);
#12419=ORIENTED_EDGE('',*,*,#9530,.F.);
#12420=ORIENTED_EDGE('',*,*,#9397,.T.);
#12421=ORIENTED_EDGE('',*,*,#9604,.F.);
#12422=ORIENTED_EDGE('',*,*,#9604,.T.);
#12423=ORIENTED_EDGE('',*,*,#9396,.T.);
#12424=ORIENTED_EDGE('',*,*,#9603,.F.);
#12425=ORIENTED_EDGE('',*,*,#9531,.T.);
#12426=ORIENTED_EDGE('',*,*,#9399,.F.);
#12427=ORIENTED_EDGE('',*,*,#9529,.T.);
#12428=ORIENTED_EDGE('',*,*,#9605,.T.);
#12429=ORIENTED_EDGE('',*,*,#9527,.F.);
#12430=ORIENTED_EDGE('',*,*,#9401,.T.);
#12431=ORIENTED_EDGE('',*,*,#9606,.F.);
#12432=ORIENTED_EDGE('',*,*,#9606,.T.);
#12433=ORIENTED_EDGE('',*,*,#9400,.T.);
#12434=ORIENTED_EDGE('',*,*,#9605,.F.);
#12435=ORIENTED_EDGE('',*,*,#9528,.T.);
#12436=ORIENTED_EDGE('',*,*,#9403,.F.);
#12437=ORIENTED_EDGE('',*,*,#9526,.T.);
#12438=ORIENTED_EDGE('',*,*,#9607,.T.);
#12439=ORIENTED_EDGE('',*,*,#9524,.F.);
#12440=ORIENTED_EDGE('',*,*,#9405,.T.);
#12441=ORIENTED_EDGE('',*,*,#9608,.F.);
#12442=ORIENTED_EDGE('',*,*,#9608,.T.);
#12443=ORIENTED_EDGE('',*,*,#9404,.T.);
#12444=ORIENTED_EDGE('',*,*,#9607,.F.);
#12445=ORIENTED_EDGE('',*,*,#9525,.T.);
#12446=ORIENTED_EDGE('',*,*,#9410,.F.);
#12447=ORIENTED_EDGE('',*,*,#9523,.T.);
#12448=ORIENTED_EDGE('',*,*,#9609,.T.);
#12449=ORIENTED_EDGE('',*,*,#9521,.F.);
#12450=ORIENTED_EDGE('',*,*,#9412,.T.);
#12451=ORIENTED_EDGE('',*,*,#9610,.F.);
#12452=ORIENTED_EDGE('',*,*,#9610,.T.);
#12453=ORIENTED_EDGE('',*,*,#9411,.T.);
#12454=ORIENTED_EDGE('',*,*,#9609,.F.);
#12455=ORIENTED_EDGE('',*,*,#9522,.T.);
#12456=ORIENTED_EDGE('',*,*,#9414,.F.);
#12457=ORIENTED_EDGE('',*,*,#9520,.T.);
#12458=ORIENTED_EDGE('',*,*,#9611,.T.);
#12459=ORIENTED_EDGE('',*,*,#9545,.F.);
#12460=ORIENTED_EDGE('',*,*,#9416,.T.);
#12461=ORIENTED_EDGE('',*,*,#9612,.F.);
#12462=ORIENTED_EDGE('',*,*,#9612,.T.);
#12463=ORIENTED_EDGE('',*,*,#9415,.T.);
#12464=ORIENTED_EDGE('',*,*,#9611,.F.);
#12465=ORIENTED_EDGE('',*,*,#9546,.T.);
#17252=TOROIDAL_SURFACE('',#18351,30.,5.);
#17253=TOROIDAL_SURFACE('',#18355,245.,5.);
#17262=ADVANCED_FACE('',(#4822),#17252,.T.);
#17263=ADVANCED_FACE('',(#4823),#17253,.T.);
#17264=ADVANCED_FACE('',(#4824),#4554,.T.);
#17265=ADVANCED_FACE('',(#4825),#4555,.F.);
#17266=ADVANCED_FACE('',(#4826),#4556,.F.);
#17267=ADVANCED_FACE('',(#4827),#4557,.F.);
#17268=ADVANCED_FACE('',(#4828),#4558,.F.);
#17269=ADVANCED_FACE('',(#4829),#4559,.F.);
#17270=ADVANCED_FACE('',(#4830),#4560,.F.);
#17271=ADVANCED_FACE('',(#4831),#4561,.F.);
#17272=ADVANCED_FACE('',(#4832),#4562,.F.);
#17273=ADVANCED_FACE('',(#4833),#4563,.T.);
#17274=ADVANCED_FACE('',(#4834),#4564,.T.);
#17275=ADVANCED_FACE('',(#4835),#4565,.F.);
#17276=ADVANCED_FACE('',(#4836),#4566,.F.);
#17277=ADVANCED_FACE('',(#4837),#4567,.F.);
#17278=ADVANCED_FACE('',(#4838),#4568,.F.);
#17279=ADVANCED_FACE('',(#4839),#4569,.F.);
#17280=ADVANCED_FACE('',(#4840),#4570,.F.);
#17281=ADVANCED_FACE('',(#4841),#4571,.F.);
#17282=ADVANCED_FACE('',(#4842),#4572,.F.);
#17283=ADVANCED_FACE('',(#4843),#4573,.F.);
#17284=ADVANCED_FACE('',(#4844),#4574,.F.);
#17285=ADVANCED_FACE('',(#4845),#4575,.F.);
#17286=ADVANCED_FACE('',(#4846),#4576,.F.);
#17287=ADVANCED_FACE('',(#4847),#4577,.F.);
#17288=ADVANCED_FACE('',(#4848),#4578,.F.);
#17289=ADVANCED_FACE('',(#4849),#4579,.F.);
#17290=ADVANCED_FACE('',(#4850),#4580,.F.);
#17291=ADVANCED_FACE('',(#4851),#4581,.F.);
#17292=ADVANCED_FACE('',(#4852),#4582,.F.);
#17293=ADVANCED_FACE('',(#4853,#876,#877),#4583,.T.);
#17294=ADVANCED_FACE('',(#4854),#4584,.T.);
#17295=ADVANCED_FACE('',(#4855,#878,#879),#4585,.F.);
#17296=ADVANCED_FACE('',(#4856,#880),#297,.T.);
#17297=ADVANCED_FACE('',(#4857,#881,#882,#883,#884,#885,#886,#887,#888,
#889,#890,#891,#892,#893,#894,#895,#896),#298,.T.);
#17298=ADVANCED_FACE('',(#4858,#897,#898,#899,#900,#901,#902,#903,#904,
#905,#906,#907,#908,#909,#910,#911,#912),#299,.F.);
#17299=ADVANCED_FACE('',(#4859,#913),#300,.F.);
#17300=ADVANCED_FACE('',(#4860,#914,#915,#916,#917,#918),#301,.T.);
#17301=ADVANCED_FACE('',(#4861,#919,#920,#921,#922,#923),#302,.F.);
#17302=ADVANCED_FACE('',(#4862),#4586,.T.);
#17303=ADVANCED_FACE('',(#4863),#303,.F.);
#17304=ADVANCED_FACE('',(#4864),#4587,.T.);
#17305=ADVANCED_FACE('',(#4865),#304,.F.);
#17306=ADVANCED_FACE('',(#4866),#4588,.T.);
#17307=ADVANCED_FACE('',(#4867),#305,.F.);
#17308=ADVANCED_FACE('',(#4868),#4589,.T.);
#17309=ADVANCED_FACE('',(#4869),#306,.F.);
#17310=ADVANCED_FACE('',(#4870,#924,#925,#926,#927,#928),#307,.T.);
#17311=ADVANCED_FACE('',(#4871,#929,#930,#931,#932,#933),#308,.F.);
#17312=ADVANCED_FACE('',(#4872),#4590,.T.);
#17313=ADVANCED_FACE('',(#4873),#309,.F.);
#17314=ADVANCED_FACE('',(#4874),#4591,.T.);
#17315=ADVANCED_FACE('',(#4875),#310,.F.);
#17316=ADVANCED_FACE('',(#4876),#4592,.T.);
#17317=ADVANCED_FACE('',(#4877),#311,.F.);
#17318=ADVANCED_FACE('',(#4878),#4593,.T.);
#17319=ADVANCED_FACE('',(#4879),#312,.F.);
#17320=ADVANCED_FACE('',(#4880,#934),#313,.T.);
#17321=ADVANCED_FACE('',(#4881),#314,.T.);
#17322=ADVANCED_FACE('',(#4882),#315,.F.);
#17323=ADVANCED_FACE('',(#4883),#316,.F.);
#17324=ADVANCED_FACE('',(#4884),#317,.T.);
#17325=ADVANCED_FACE('',(#4885),#318,.F.);
#17326=ADVANCED_FACE('',(#4886),#319,.F.);
#17327=ADVANCED_FACE('',(#4887),#320,.T.);
#17328=ADVANCED_FACE('',(#4888),#321,.F.);
#17329=ADVANCED_FACE('',(#4889),#322,.F.);
#17330=ADVANCED_FACE('',(#4890),#323,.T.);
#17331=ADVANCED_FACE('',(#4891),#324,.F.);
#17332=ADVANCED_FACE('',(#4892),#325,.F.);
#17333=ADVANCED_FACE('',(#4893),#326,.T.);
#17334=ADVANCED_FACE('',(#4894),#327,.F.);
#17335=ADVANCED_FACE('',(#4895),#328,.F.);
#17336=ADVANCED_FACE('',(#4896),#329,.T.);
#17337=ADVANCED_FACE('',(#4897),#330,.F.);
#17338=ADVANCED_FACE('',(#4898),#331,.F.);
#17339=ADVANCED_FACE('',(#4899),#332,.T.);
#17340=ADVANCED_FACE('',(#4900),#333,.F.);
#17341=ADVANCED_FACE('',(#4901),#334,.F.);
#17342=ADVANCED_FACE('',(#4902),#335,.T.);
#17343=ADVANCED_FACE('',(#4903),#336,.F.);
#17344=ADVANCED_FACE('',(#4904),#337,.F.);
#17345=ADVANCED_FACE('',(#4905),#338,.T.);
#17346=ADVANCED_FACE('',(#4906),#339,.F.);
#17347=ADVANCED_FACE('',(#4907),#340,.F.);
#18259=CLOSED_SHELL('',(#17262,#17263,#17264,#17265,#17266,#17267,#17268,
#17269,#17270,#17271,#17272,#17273,#17274,#17275,#17276,#17277,#17278,#17279,
#17280,#17281,#17282,#17283,#17284,#17285,#17286,#17287,#17288,#17289,#17290,
#17291,#17292,#17293,#17294,#17295,#17296,#17297,#17298,#17299,#17300,#17301,
#17302,#17303,#17304,#17305,#17306,#17307,#17308,#17309,#17310,#17311,#17312,
#17313,#17314,#17315,#17316,#17317,#17318,#17319,#17320,#17321,#17322,#17323,
#17324,#17325,#17326,#17327,#17328,#17329,#17330,#17331,#17332,#17333,#17334,
#17335,#17336,#17337,#17338,#17339,#17340,#17341,#17342,#17343,#17344,#17345,
#17346,#17347));
#18350=AXIS2_PLACEMENT_3D('',#24906,#20012,#20013);
#18351=AXIS2_PLACEMENT_3D('',#24907,#20014,#20015);
#18352=AXIS2_PLACEMENT_3D('',#24909,#20016,#20017);
#18353=AXIS2_PLACEMENT_3D('',#24911,#20018,#20019);
#18354=AXIS2_PLACEMENT_3D('',#24912,#20020,#20021);
#18355=AXIS2_PLACEMENT_3D('',#24913,#20022,#20023);
#18356=AXIS2_PLACEMENT_3D('',#24916,#20024,#20025);
#18357=AXIS2_PLACEMENT_3D('',#24917,#20026,#20027);
#18358=AXIS2_PLACEMENT_3D('',#24919,#20028,#20029);
#18359=AXIS2_PLACEMENT_3D('',#24920,#20030,#20031);
#18360=AXIS2_PLACEMENT_3D('',#24921,#20032,#20033);
#18361=AXIS2_PLACEMENT_3D('',#24924,#20034,#20035);
#18362=AXIS2_PLACEMENT_3D('',#24928,#20037,#20038);
#18363=AXIS2_PLACEMENT_3D('',#24932,#20040,#20041);
#18364=AXIS2_PLACEMENT_3D('',#24936,#20043,#20044);
#18365=AXIS2_PLACEMENT_3D('',#24940,#20046,#20047);
#18366=AXIS2_PLACEMENT_3D('',#24944,#20049,#20050);
#18367=AXIS2_PLACEMENT_3D('',#24948,#20052,#20053);
#18368=AXIS2_PLACEMENT_3D('',#24952,#20055,#20056);
#18369=AXIS2_PLACEMENT_3D('',#24956,#20058,#20059);
#18370=AXIS2_PLACEMENT_3D('',#24959,#20061,#20062);
#18371=AXIS2_PLACEMENT_3D('',#24961,#20063,#20064);
#18372=AXIS2_PLACEMENT_3D('',#24965,#20066,#20067);
#18373=AXIS2_PLACEMENT_3D('',#24969,#20069,#20070);
#18374=AXIS2_PLACEMENT_3D('',#24973,#20072,#20073);
#18375=AXIS2_PLACEMENT_3D('',#24977,#20075,#20076);
#18376=AXIS2_PLACEMENT_3D('',#24981,#20078,#20079);
#18377=AXIS2_PLACEMENT_3D('',#24985,#20081,#20082);
#18378=AXIS2_PLACEMENT_3D('',#24989,#20084,#20085);
#18379=AXIS2_PLACEMENT_3D('',#24993,#20087,#20088);
#18380=AXIS2_PLACEMENT_3D('',#24997,#20090,#20091);
#18381=AXIS2_PLACEMENT_3D('',#24999,#20093,#20094);
#18382=AXIS2_PLACEMENT_3D('',#25001,#20095,#20096);
#18383=AXIS2_PLACEMENT_3D('',#25004,#20098,#20099);
#18384=AXIS2_PLACEMENT_3D('',#25005,#20100,#20101);
#18385=AXIS2_PLACEMENT_3D('',#25007,#20102,#20103);
#18386=AXIS2_PLACEMENT_3D('',#25010,#20105,#20106);
#18387=AXIS2_PLACEMENT_3D('',#25011,#20107,#20108);
#18388=AXIS2_PLACEMENT_3D('',#25013,#20109,#20110);
#18389=AXIS2_PLACEMENT_3D('',#25016,#20112,#20113);
#18390=AXIS2_PLACEMENT_3D('',#25017,#20114,#20115);
#18391=AXIS2_PLACEMENT_3D('',#25019,#20116,#20117);
#18392=AXIS2_PLACEMENT_3D('',#25022,#20119,#20120);
#18393=AXIS2_PLACEMENT_3D('',#25023,#20121,#20122);
#18394=AXIS2_PLACEMENT_3D('',#25025,#20123,#20124);
#18395=AXIS2_PLACEMENT_3D('',#25028,#20126,#20127);
#18396=AXIS2_PLACEMENT_3D('',#25029,#20128,#20129);
#18397=AXIS2_PLACEMENT_3D('',#25031,#20130,#20131);
#18398=AXIS2_PLACEMENT_3D('',#25034,#20133,#20134);
#18399=AXIS2_PLACEMENT_3D('',#25035,#20135,#20136);
#18400=AXIS2_PLACEMENT_3D('',#25037,#20137,#20138);
#18401=AXIS2_PLACEMENT_3D('',#25040,#20140,#20141);
#18402=AXIS2_PLACEMENT_3D('',#25041,#20142,#20143);
#18403=AXIS2_PLACEMENT_3D('',#25043,#20144,#20145);
#18404=AXIS2_PLACEMENT_3D('',#25046,#20147,#20148);
#18405=AXIS2_PLACEMENT_3D('',#25047,#20149,#20150);
#18406=AXIS2_PLACEMENT_3D('',#25113,#20152,#20153);
#18407=AXIS2_PLACEMENT_3D('',#25114,#20154,#20155);
#18408=AXIS2_PLACEMENT_3D('',#25180,#20157,#20158);
#18409=AXIS2_PLACEMENT_3D('',#25181,#20159,#20160);
#18410=AXIS2_PLACEMENT_3D('',#25251,#20162,#20163);
#18411=AXIS2_PLACEMENT_3D('',#25252,#20164,#20165);
#18412=AXIS2_PLACEMENT_3D('',#25322,#20167,#20168);
#18413=AXIS2_PLACEMENT_3D('',#25323,#20169,#20170);
#18414=AXIS2_PLACEMENT_3D('',#25326,#20172,#20173);
#18415=AXIS2_PLACEMENT_3D('',#25327,#20174,#20175);
#18416=AXIS2_PLACEMENT_3D('',#25329,#20176,#20177);
#18417=AXIS2_PLACEMENT_3D('',#25332,#20179,#20180);
#18418=AXIS2_PLACEMENT_3D('',#25333,#20181,#20182);
#18419=AXIS2_PLACEMENT_3D('',#25335,#20183,#20184);
#18420=AXIS2_PLACEMENT_3D('',#25338,#20186,#20187);
#18421=AXIS2_PLACEMENT_3D('',#25339,#20188,#20189);
#18422=AXIS2_PLACEMENT_3D('',#25341,#20190,#20191);
#18423=AXIS2_PLACEMENT_3D('',#25344,#20193,#20194);
#18424=AXIS2_PLACEMENT_3D('',#25345,#20195,#20196);
#18425=AXIS2_PLACEMENT_3D('',#25347,#20197,#20198);
#18426=AXIS2_PLACEMENT_3D('',#25350,#20200,#20201);
#18427=AXIS2_PLACEMENT_3D('',#25351,#20202,#20203);
#18428=AXIS2_PLACEMENT_3D('',#25353,#20204,#20205);
#18429=AXIS2_PLACEMENT_3D('',#25356,#20207,#20208);
#18430=AXIS2_PLACEMENT_3D('',#25357,#20209,#20210);
#18431=AXIS2_PLACEMENT_3D('',#25359,#20211,#20212);
#18432=AXIS2_PLACEMENT_3D('',#25362,#20214,#20215);
#18433=AXIS2_PLACEMENT_3D('',#25363,#20216,#20217);
#18434=AXIS2_PLACEMENT_3D('',#25365,#20218,#20219);
#18435=AXIS2_PLACEMENT_3D('',#25368,#20221,#20222);
#18436=AXIS2_PLACEMENT_3D('',#25369,#20223,#20224);
#18437=AXIS2_PLACEMENT_3D('',#25371,#20225,#20226);
#18438=AXIS2_PLACEMENT_3D('',#25374,#20228,#20229);
#18439=AXIS2_PLACEMENT_3D('',#25375,#20230,#20231);
#18440=AXIS2_PLACEMENT_3D('',#25377,#20232,#20233);
#18441=AXIS2_PLACEMENT_3D('',#25380,#20235,#20236);
#18442=AXIS2_PLACEMENT_3D('',#25381,#20237,#20238);
#18443=AXIS2_PLACEMENT_3D('',#25383,#20239,#20240);
#18444=AXIS2_PLACEMENT_3D('',#25386,#20242,#20243);
#18445=AXIS2_PLACEMENT_3D('',#25387,#20244,#20245);
#18446=AXIS2_PLACEMENT_3D('',#25389,#20246,#20247);
#18447=AXIS2_PLACEMENT_3D('',#25392,#20249,#20250);
#18448=AXIS2_PLACEMENT_3D('',#25393,#20251,#20252);
#18449=AXIS2_PLACEMENT_3D('',#25395,#20253,#20254);
#18450=AXIS2_PLACEMENT_3D('',#25398,#20256,#20257);
#18451=AXIS2_PLACEMENT_3D('',#25399,#20258,#20259);
#18452=AXIS2_PLACEMENT_3D('',#25401,#20260,#20261);
#18453=AXIS2_PLACEMENT_3D('',#25404,#20263,#20264);
#18454=AXIS2_PLACEMENT_3D('',#25405,#20265,#20266);
#18455=AXIS2_PLACEMENT_3D('',#25407,#20267,#20268);
#18456=AXIS2_PLACEMENT_3D('',#25410,#20270,#20271);
#18457=AXIS2_PLACEMENT_3D('',#25411,#20272,#20273);
#18458=AXIS2_PLACEMENT_3D('',#25413,#20274,#20275);
#18459=AXIS2_PLACEMENT_3D('',#25416,#20277,#20278);
#18460=AXIS2_PLACEMENT_3D('',#25417,#20279,#20280);
#18461=AXIS2_PLACEMENT_3D('',#25420,#20282,#20283);
#18462=AXIS2_PLACEMENT_3D('',#25421,#20284,#20285);
#18463=AXIS2_PLACEMENT_3D('',#25423,#20286,#20287);
#18464=AXIS2_PLACEMENT_3D('',#25426,#20289,#20290);
#18465=AXIS2_PLACEMENT_3D('',#25427,#20291,#20292);
#18466=AXIS2_PLACEMENT_3D('',#25429,#20293,#20294);
#18467=AXIS2_PLACEMENT_3D('',#25432,#20296,#20297);
#18468=AXIS2_PLACEMENT_3D('',#25433,#20298,#20299);
#18469=AXIS2_PLACEMENT_3D('',#25479,#20327,#20328);
#18470=AXIS2_PLACEMENT_3D('',#25480,#20329,#20330);
#18471=AXIS2_PLACEMENT_3D('',#25481,#20331,#20332);
#18472=AXIS2_PLACEMENT_3D('',#25482,#20333,#20334);
#18473=AXIS2_PLACEMENT_3D('',#25485,#20335,#20336);
#18474=AXIS2_PLACEMENT_3D('',#25489,#20338,#20339);
#18475=AXIS2_PLACEMENT_3D('',#25493,#20341,#20342);
#18476=AXIS2_PLACEMENT_3D('',#25497,#20344,#20345);
#18477=AXIS2_PLACEMENT_3D('',#25499,#20347,#20348);
#18478=AXIS2_PLACEMENT_3D('',#25502,#20349,#20350);
#18479=AXIS2_PLACEMENT_3D('',#25506,#20352,#20353);
#18480=AXIS2_PLACEMENT_3D('',#25510,#20355,#20356);
#18481=AXIS2_PLACEMENT_3D('',#25514,#20358,#20359);
#18482=AXIS2_PLACEMENT_3D('',#25516,#20361,#20362);
#18483=AXIS2_PLACEMENT_3D('',#25519,#20365,#20366);
#18484=AXIS2_PLACEMENT_3D('',#25521,#20368,#20369);
#18485=AXIS2_PLACEMENT_3D('',#25523,#20371,#20372);
#18486=AXIS2_PLACEMENT_3D('',#25525,#20374,#20375);
#18487=AXIS2_PLACEMENT_3D('',#25527,#20377,#20378);
#18488=AXIS2_PLACEMENT_3D('',#25529,#20380,#20381);
#18489=AXIS2_PLACEMENT_3D('',#25531,#20383,#20384);
#18490=AXIS2_PLACEMENT_3D('',#25532,#20385,#20386);
#18491=AXIS2_PLACEMENT_3D('',#25535,#20387,#20388);
#18492=AXIS2_PLACEMENT_3D('',#25539,#20390,#20391);
#18493=AXIS2_PLACEMENT_3D('',#25543,#20393,#20394);
#18494=AXIS2_PLACEMENT_3D('',#25547,#20396,#20397);
#18495=AXIS2_PLACEMENT_3D('',#25549,#20399,#20400);
#18496=AXIS2_PLACEMENT_3D('',#25552,#20401,#20402);
#18497=AXIS2_PLACEMENT_3D('',#25556,#20404,#20405);
#18498=AXIS2_PLACEMENT_3D('',#25560,#20407,#20408);
#18499=AXIS2_PLACEMENT_3D('',#25564,#20410,#20411);
#18500=AXIS2_PLACEMENT_3D('',#25566,#20413,#20414);
#18501=AXIS2_PLACEMENT_3D('',#25569,#20417,#20418);
#18502=AXIS2_PLACEMENT_3D('',#25571,#20420,#20421);
#18503=AXIS2_PLACEMENT_3D('',#25573,#20423,#20424);
#18504=AXIS2_PLACEMENT_3D('',#25575,#20426,#20427);
#18505=AXIS2_PLACEMENT_3D('',#25577,#20429,#20430);
#18506=AXIS2_PLACEMENT_3D('',#25579,#20432,#20433);
#18507=AXIS2_PLACEMENT_3D('',#25581,#20435,#20436);
#18508=AXIS2_PLACEMENT_3D('',#25582,#20437,#20438);
#18509=AXIS2_PLACEMENT_3D('',#25583,#20439,#20440);
#18510=AXIS2_PLACEMENT_3D('',#25585,#20442,#20443);
#18511=AXIS2_PLACEMENT_3D('',#25587,#20445,#20446);
#18512=AXIS2_PLACEMENT_3D('',#25588,#20447,#20448);
#18513=AXIS2_PLACEMENT_3D('',#25590,#20450,#20451);
#18514=AXIS2_PLACEMENT_3D('',#25592,#20453,#20454);
#18515=AXIS2_PLACEMENT_3D('',#25593,#20455,#20456);
#18516=AXIS2_PLACEMENT_3D('',#25595,#20458,#20459);
#18517=AXIS2_PLACEMENT_3D('',#25597,#20461,#20462);
#18518=AXIS2_PLACEMENT_3D('',#25598,#20463,#20464);
#18519=AXIS2_PLACEMENT_3D('',#25600,#20466,#20467);
#18520=AXIS2_PLACEMENT_3D('',#25602,#20469,#20470);
#18521=AXIS2_PLACEMENT_3D('',#25603,#20471,#20472);
#18522=AXIS2_PLACEMENT_3D('',#25605,#20474,#20475);
#18523=AXIS2_PLACEMENT_3D('',#25607,#20477,#20478);
#18524=AXIS2_PLACEMENT_3D('',#25608,#20479,#20480);
#18525=AXIS2_PLACEMENT_3D('',#25610,#20482,#20483);
#18526=AXIS2_PLACEMENT_3D('',#25612,#20485,#20486);
#18527=AXIS2_PLACEMENT_3D('',#25613,#20487,#20488);
#18528=AXIS2_PLACEMENT_3D('',#25615,#20490,#20491);
#18529=AXIS2_PLACEMENT_3D('',#25617,#20493,#20494);
#18530=AXIS2_PLACEMENT_3D('',#25618,#20495,#20496);
#18531=AXIS2_PLACEMENT_3D('',#25620,#20498,#20499);
#18532=AXIS2_PLACEMENT_3D('',#25622,#20501,#20502);
#18533=AXIS2_PLACEMENT_3D('',#25623,#20503,#20504);
#18534=AXIS2_PLACEMENT_3D('',#25625,#20506,#20507);
#18535=AXIS2_PLACEMENT_3D('',#25627,#20509,#20510);
#20012=DIRECTION('axis',(0.,0.,1.));
#20013=DIRECTION('refdir',(1.,0.,0.));
#20014=DIRECTION('center_axis',(0.,0.,1.));
#20015=DIRECTION('ref_axis',(1.,0.,0.));
#20016=DIRECTION('center_axis',(0.,0.,1.));
#20017=DIRECTION('ref_axis',(1.,0.,0.));
#20018=DIRECTION('center_axis',(1.22464679914735E-16,-1.,0.));
#20019=DIRECTION('ref_axis',(-1.,-1.22464679914735E-16,0.));
#20020=DIRECTION('center_axis',(0.,0.,-1.));
#20021=DIRECTION('ref_axis',(1.,0.,0.));
#20022=DIRECTION('center_axis',(0.,0.,1.));
#20023=DIRECTION('ref_axis',(1.,0.,0.));
#20024=DIRECTION('center_axis',(0.,0.,1.));
#20025=DIRECTION('ref_axis',(1.,0.,0.));
#20026=DIRECTION('center_axis',(0.,0.,1.));
#20027=DIRECTION('ref_axis',(1.,0.,0.));
#20028=DIRECTION('center_axis',(1.22464679914735E-16,-1.,0.));
#20029=DIRECTION('ref_axis',(-1.,-1.22464679914735E-16,0.));
#20030=DIRECTION('center_axis',(0.,0.,-1.));
#20031=DIRECTION('ref_axis',(1.,0.,0.));
#20032=DIRECTION('center_axis',(0.,0.,-1.));
#20033=DIRECTION('ref_axis',(-1.,0.,0.));
#20034=DIRECTION('center_axis',(0.,0.,1.));
#20035=DIRECTION('ref_axis',(1.,0.,0.));
#20036=DIRECTION('',(0.,0.,1.));
#20037=DIRECTION('center_axis',(0.255411479413649,0.147461886393592,-0.955520783784934));
#20038=DIRECTION('ref_axis',(-0.827505272601769,-0.47776039189247,-0.294923772787182));
#20039=DIRECTION('',(0.,0.,1.));
#20040=DIRECTION('center_axis',(0.,0.,1.));
#20041=DIRECTION('ref_axis',(1.,0.,0.));
#20042=DIRECTION('',(0.,0.,1.));
#20043=DIRECTION('center_axis',(0.100869871038817,0.277137692982455,-0.955520783784934));
#20044=DIRECTION('ref_axis',(-0.326807355420773,-0.897895829530272,-0.294923772787182));
#20045=DIRECTION('',(0.,0.,1.));
#20046=DIRECTION('center_axis',(0.,0.,1.));
#20047=DIRECTION('ref_axis',(1.,0.,0.));
#20048=DIRECTION('',(0.,0.,1.));
#20049=DIRECTION('center_axis',(-0.100869871038821,0.277137692982454,-0.955520783784934));
#20050=DIRECTION('ref_axis',(-0.326807355420785,0.897895829530268,0.294923772787182));
#20051=DIRECTION('',(0.,0.,1.));
#20052=DIRECTION('center_axis',(0.,0.,1.));
#20053=DIRECTION('ref_axis',(1.,0.,0.));
#20054=DIRECTION('',(0.,0.,1.));
#20055=DIRECTION('center_axis',(-0.255411479413651,0.147461886393589,-0.955520783784934));
#20056=DIRECTION('ref_axis',(-0.827505272601775,0.47776039189246,0.294923772787182));
#20057=DIRECTION('',(0.,0.,1.));
#20058=DIRECTION('center_axis',(0.,0.,1.));
#20059=DIRECTION('ref_axis',(1.,0.,0.));
#20060=DIRECTION('',(0.,0.,1.));
#20061=DIRECTION('center_axis',(0.,0.,1.));
#20062=DIRECTION('ref_axis',(1.,0.,0.));
#20063=DIRECTION('center_axis',(0.,0.,1.));
#20064=DIRECTION('ref_axis',(1.,0.,0.));
#20065=DIRECTION('',(0.,0.,1.));
#20066=DIRECTION('center_axis',(-0.290443217988427,-0.0512129756951529,
-0.955520783784934));
#20067=DIRECTION('ref_axis',(-0.941004276035703,-0.165924442827141,0.294923772787182));
#20068=DIRECTION('',(0.,0.,1.));
#20069=DIRECTION('center_axis',(0.,0.,1.));
#20070=DIRECTION('ref_axis',(1.,0.,0.));
#20071=DIRECTION('',(0.,0.,1.));
#20072=DIRECTION('center_axis',(-0.189573346949606,-0.225924717287307,-0.955520783784934));
#20073=DIRECTION('ref_axis',(-0.614196920614917,-0.731971386703147,0.294923772787182));
#20074=DIRECTION('',(0.,0.,1.));
#20075=DIRECTION('center_axis',(0.,0.,1.));
#20076=DIRECTION('ref_axis',(1.,0.,0.));
#20077=DIRECTION('',(0.,0.,1.));
#20078=DIRECTION('center_axis',(0.,-0.294923772787182,-0.955520783784934));
#20079=DIRECTION('ref_axis',(0.,0.955520783784934,-0.294923772787182));
#20080=DIRECTION('',(0.,0.,1.));
#20081=DIRECTION('center_axis',(0.,0.,1.));
#20082=DIRECTION('ref_axis',(1.,0.,0.));
#20083=DIRECTION('',(0.,0.,1.));
#20084=DIRECTION('center_axis',(0.189573346949609,-0.225924717287304,-0.955520783784934));
#20085=DIRECTION('ref_axis',(-0.614196920614927,0.731971386703139,-0.294923772787182));
#20086=DIRECTION('',(0.,0.,1.));
#20087=DIRECTION('center_axis',(0.,0.,1.));
#20088=DIRECTION('ref_axis',(1.,0.,0.));
#20089=DIRECTION('',(0.,0.,1.));
#20090=DIRECTION('center_axis',(0.290443217988428,-0.0512129756951491,-0.955520783784934));
#20091=DIRECTION('ref_axis',(-0.941004276035705,0.165924442827128,-0.294923772787182));
#20092=DIRECTION('',(0.,0.,1.));
#20093=DIRECTION('center_axis',(-1.,-1.26189474349424E-16,0.));
#20094=DIRECTION('ref_axis',(1.26189474349424E-16,-1.,0.));
#20095=DIRECTION('center_axis',(1.,1.26189474349424E-16,0.));
#20096=DIRECTION('ref_axis',(1.26189474349424E-16,-1.,0.));
#20097=DIRECTION('',(-1.,-1.26189474349424E-16,0.));
#20098=DIRECTION('center_axis',(1.,1.26189474349424E-16,0.));
#20099=DIRECTION('ref_axis',(1.26189474349424E-16,-1.,0.));
#20100=DIRECTION('center_axis',(-1.,-1.26189474349424E-16,0.));
#20101=DIRECTION('ref_axis',(1.26189474349424E-16,-1.,0.));
#20102=DIRECTION('center_axis',(1.,1.26189474349424E-16,0.));
#20103=DIRECTION('ref_axis',(-1.26189474349424E-16,1.,0.));
#20104=DIRECTION('',(-1.,-1.26189474349424E-16,0.));
#20105=DIRECTION('center_axis',(1.,1.26189474349424E-16,0.));
#20106=DIRECTION('ref_axis',(-1.26189474349424E-16,1.,0.));
#20107=DIRECTION('center_axis',(-1.,-1.26189474349424E-16,0.));
#20108=DIRECTION('ref_axis',(1.26189474349424E-16,-1.,0.));
#20109=DIRECTION('center_axis',(1.,1.26189474349424E-16,0.));
#20110=DIRECTION('ref_axis',(1.26189474349424E-16,-1.,0.));
#20111=DIRECTION('',(-1.,-1.26189474349424E-16,0.));
#20112=DIRECTION('center_axis',(1.,1.26189474349424E-16,0.));
#20113=DIRECTION('ref_axis',(1.26189474349424E-16,-1.,0.));
#20114=DIRECTION('center_axis',(-1.,-1.26189474349424E-16,0.));
#20115=DIRECTION('ref_axis',(1.26189474349424E-16,-1.,0.));
#20116=DIRECTION('center_axis',(1.,1.26189474349424E-16,0.));
#20117=DIRECTION('ref_axis',(-1.26189474349424E-16,1.,0.));
#20118=DIRECTION('',(-1.,-1.26189474349424E-16,0.));
#20119=DIRECTION('center_axis',(1.,1.26189474349424E-16,0.));
#20120=DIRECTION('ref_axis',(-1.26189474349424E-16,1.,0.));
#20121=DIRECTION('center_axis',(-1.,-1.26189474349424E-16,0.));
#20122=DIRECTION('ref_axis',(1.26189474349424E-16,-1.,0.));
#20123=DIRECTION('center_axis',(1.,1.26189474349424E-16,0.));
#20124=DIRECTION('ref_axis',(1.26189474349424E-16,-1.,0.));
#20125=DIRECTION('',(-1.,-1.26189474349424E-16,0.));
#20126=DIRECTION('center_axis',(1.,1.26189474349424E-16,0.));
#20127=DIRECTION('ref_axis',(1.26189474349424E-16,-1.,0.));
#20128=DIRECTION('center_axis',(-1.,-1.26189474349424E-16,0.));
#20129=DIRECTION('ref_axis',(1.26189474349424E-16,-1.,0.));
#20130=DIRECTION('center_axis',(1.,1.26189474349424E-16,0.));
#20131=DIRECTION('ref_axis',(1.26189474349424E-16,-1.,0.));
#20132=DIRECTION('',(-1.,-1.26189474349424E-16,0.));
#20133=DIRECTION('center_axis',(1.,1.26189474349424E-16,0.));
#20134=DIRECTION('ref_axis',(1.26189474349424E-16,-1.,0.));
#20135=DIRECTION('center_axis',(-1.,-1.26189474349424E-16,0.));
#20136=DIRECTION('ref_axis',(1.26189474349424E-16,-1.,0.));
#20137=DIRECTION('center_axis',(1.,1.26189474349424E-16,0.));
#20138=DIRECTION('ref_axis',(-1.26189474349424E-16,1.,0.));
#20139=DIRECTION('',(-1.,-1.26189474349424E-16,0.));
#20140=DIRECTION('center_axis',(1.,1.26189474349424E-16,0.));
#20141=DIRECTION('ref_axis',(-1.26189474349424E-16,1.,0.));
#20142=DIRECTION('center_axis',(-1.,-1.26189474349424E-16,0.));
#20143=DIRECTION('ref_axis',(1.26189474349424E-16,-1.,0.));
#20144=DIRECTION('center_axis',(1.,1.26189474349424E-16,0.));
#20145=DIRECTION('ref_axis',(-1.26189474349424E-16,1.,0.));
#20146=DIRECTION('',(-1.,-1.26189474349424E-16,0.));
#20147=DIRECTION('center_axis',(1.,1.26189474349424E-16,0.));
#20148=DIRECTION('ref_axis',(-1.26189474349424E-16,1.,0.));
#20149=DIRECTION('center_axis',(-1.,-1.26189474349424E-16,0.));
#20150=DIRECTION('ref_axis',(1.26189474349424E-16,-1.,0.));
#20151=DIRECTION('',(1.,1.26189474349424E-16,0.));
#20152=DIRECTION('center_axis',(-1.,-1.26189474349424E-16,0.));
#20153=DIRECTION('ref_axis',(1.26189474349424E-16,-1.,0.));
#20154=DIRECTION('center_axis',(-1.,-1.26189474349424E-16,0.));
#20155=DIRECTION('ref_axis',(1.26189474349424E-16,-1.,0.));
#20156=DIRECTION('',(1.,1.26189474349424E-16,0.));
#20157=DIRECTION('center_axis',(-1.,-1.26189474349424E-16,0.));
#20158=DIRECTION('ref_axis',(-1.26189474349424E-16,1.,0.));
#20159=DIRECTION('center_axis',(1.,-3.84524791680814E-16,0.));
#20160=DIRECTION('ref_axis',(-3.84524791680814E-16,-1.,0.));
#20161=DIRECTION('',(1.,-3.84524791680814E-16,0.));
#20162=DIRECTION('center_axis',(1.,1.26189474349424E-16,0.));
#20163=DIRECTION('ref_axis',(1.26189474349424E-16,-1.,0.));
#20164=DIRECTION('center_axis',(1.,3.84524791680814E-16,0.));
#20165=DIRECTION('ref_axis',(-3.84524791680814E-16,1.,0.));
#20166=DIRECTION('',(1.,3.84524791680814E-16,0.));
#20167=DIRECTION('center_axis',(1.,1.26189474349424E-16,0.));
#20168=DIRECTION('ref_axis',(-1.26189474349424E-16,1.,0.));
#20169=DIRECTION('center_axis',(0.,0.,1.));
#20170=DIRECTION('ref_axis',(1.,0.,0.));
#20171=DIRECTION('',(0.,0.,1.));
#20172=DIRECTION('center_axis',(0.,0.,1.));
#20173=DIRECTION('ref_axis',(1.,0.,0.));
#20174=DIRECTION('center_axis',(0.,0.,1.));
#20175=DIRECTION('ref_axis',(1.,0.,0.));
#20176=DIRECTION('center_axis',(0.,0.,1.));
#20177=DIRECTION('ref_axis',(1.,0.,0.));
#20178=DIRECTION('',(0.,0.,1.));
#20179=DIRECTION('center_axis',(0.,0.,1.));
#20180=DIRECTION('ref_axis',(1.,0.,0.));
#20181=DIRECTION('center_axis',(0.,0.,1.));
#20182=DIRECTION('ref_axis',(1.,0.,0.));
#20183=DIRECTION('center_axis',(0.,0.,1.));
#20184=DIRECTION('ref_axis',(1.,0.,0.));
#20185=DIRECTION('',(0.,0.,1.));
#20186=DIRECTION('center_axis',(0.,0.,1.));
#20187=DIRECTION('ref_axis',(1.,0.,0.));
#20188=DIRECTION('center_axis',(0.,0.,1.));
#20189=DIRECTION('ref_axis',(1.,0.,0.));
#20190=DIRECTION('center_axis',(0.,0.,1.));
#20191=DIRECTION('ref_axis',(1.,0.,0.));
#20192=DIRECTION('',(0.,0.,1.));
#20193=DIRECTION('center_axis',(0.,0.,1.));
#20194=DIRECTION('ref_axis',(1.,0.,0.));
#20195=DIRECTION('center_axis',(0.,0.,1.));
#20196=DIRECTION('ref_axis',(1.,0.,0.));
#20197=DIRECTION('center_axis',(0.,0.,1.));
#20198=DIRECTION('ref_axis',(1.,0.,0.));
#20199=DIRECTION('',(0.,0.,1.));
#20200=DIRECTION('center_axis',(0.,0.,1.));
#20201=DIRECTION('ref_axis',(1.,0.,0.));
#20202=DIRECTION('center_axis',(0.,0.,1.));
#20203=DIRECTION('ref_axis',(1.,0.,0.));
#20204=DIRECTION('center_axis',(0.,0.,1.));
#20205=DIRECTION('ref_axis',(1.,0.,0.));
#20206=DIRECTION('',(0.,0.,1.));
#20207=DIRECTION('center_axis',(0.,0.,1.));
#20208=DIRECTION('ref_axis',(1.,0.,0.));
#20209=DIRECTION('center_axis',(0.,0.,1.));
#20210=DIRECTION('ref_axis',(1.,0.,0.));
#20211=DIRECTION('center_axis',(0.,0.,1.));
#20212=DIRECTION('ref_axis',(1.,0.,0.));
#20213=DIRECTION('',(0.,0.,1.));
#20214=DIRECTION('center_axis',(0.,0.,1.));
#20215=DIRECTION('ref_axis',(1.,0.,0.));
#20216=DIRECTION('center_axis',(0.,0.,1.));
#20217=DIRECTION('ref_axis',(1.,0.,0.));
#20218=DIRECTION('center_axis',(0.,0.,1.));
#20219=DIRECTION('ref_axis',(1.,0.,0.));
#20220=DIRECTION('',(0.,0.,1.));
#20221=DIRECTION('center_axis',(0.,0.,1.));
#20222=DIRECTION('ref_axis',(1.,0.,0.));
#20223=DIRECTION('center_axis',(0.,0.,1.));
#20224=DIRECTION('ref_axis',(1.,0.,0.));
#20225=DIRECTION('center_axis',(0.,0.,1.));
#20226=DIRECTION('ref_axis',(1.,0.,0.));
#20227=DIRECTION('',(0.,0.,1.));
#20228=DIRECTION('center_axis',(0.,0.,1.));
#20229=DIRECTION('ref_axis',(1.,0.,0.));
#20230=DIRECTION('center_axis',(0.,0.,1.));
#20231=DIRECTION('ref_axis',(1.,0.,0.));
#20232=DIRECTION('center_axis',(0.,0.,1.));
#20233=DIRECTION('ref_axis',(1.,0.,0.));
#20234=DIRECTION('',(0.,0.,1.));
#20235=DIRECTION('center_axis',(0.,0.,1.));
#20236=DIRECTION('ref_axis',(1.,0.,0.));
#20237=DIRECTION('center_axis',(0.,0.,1.));
#20238=DIRECTION('ref_axis',(1.,0.,0.));
#20239=DIRECTION('center_axis',(0.,0.,1.));
#20240=DIRECTION('ref_axis',(1.,0.,0.));
#20241=DIRECTION('',(0.,0.,1.));
#20242=DIRECTION('center_axis',(0.,0.,1.));
#20243=DIRECTION('ref_axis',(1.,0.,0.));
#20244=DIRECTION('center_axis',(0.,0.,1.));
#20245=DIRECTION('ref_axis',(1.,0.,0.));
#20246=DIRECTION('center_axis',(0.,0.,1.));
#20247=DIRECTION('ref_axis',(1.,0.,0.));
#20248=DIRECTION('',(0.,0.,1.));
#20249=DIRECTION('center_axis',(0.,0.,1.));
#20250=DIRECTION('ref_axis',(1.,0.,0.));
#20251=DIRECTION('center_axis',(0.,0.,1.));
#20252=DIRECTION('ref_axis',(1.,0.,0.));
#20253=DIRECTION('center_axis',(0.,0.,1.));
#20254=DIRECTION('ref_axis',(1.,0.,0.));
#20255=DIRECTION('',(0.,0.,1.));
#20256=DIRECTION('center_axis',(0.,0.,1.));
#20257=DIRECTION('ref_axis',(1.,0.,0.));
#20258=DIRECTION('center_axis',(0.,0.,1.));
#20259=DIRECTION('ref_axis',(1.,0.,0.));
#20260=DIRECTION('center_axis',(0.,0.,1.));
#20261=DIRECTION('ref_axis',(1.,0.,0.));
#20262=DIRECTION('',(0.,0.,1.));
#20263=DIRECTION('center_axis',(0.,0.,1.));
#20264=DIRECTION('ref_axis',(1.,0.,0.));
#20265=DIRECTION('center_axis',(0.,0.,1.));
#20266=DIRECTION('ref_axis',(1.,0.,0.));
#20267=DIRECTION('center_axis',(0.,0.,1.));
#20268=DIRECTION('ref_axis',(1.,0.,0.));
#20269=DIRECTION('',(0.,0.,1.));
#20270=DIRECTION('center_axis',(0.,0.,1.));
#20271=DIRECTION('ref_axis',(1.,0.,0.));
#20272=DIRECTION('center_axis',(0.,0.,1.));
#20273=DIRECTION('ref_axis',(1.,0.,0.));
#20274=DIRECTION('center_axis',(0.,0.,1.));
#20275=DIRECTION('ref_axis',(1.,0.,0.));
#20276=DIRECTION('',(0.,0.,1.));
#20277=DIRECTION('center_axis',(0.,0.,1.));
#20278=DIRECTION('ref_axis',(1.,0.,0.));
#20279=DIRECTION('center_axis',(0.,0.,-1.));
#20280=DIRECTION('ref_axis',(-1.,0.,0.));
#20281=DIRECTION('',(0.,0.,1.));
#20282=DIRECTION('center_axis',(0.,0.,1.));
#20283=DIRECTION('ref_axis',(1.,0.,0.));
#20284=DIRECTION('center_axis',(0.,0.,1.));
#20285=DIRECTION('ref_axis',(1.,0.,0.));
#20286=DIRECTION('center_axis',(0.,0.,1.));
#20287=DIRECTION('ref_axis',(1.,0.,0.));
#20288=DIRECTION('',(0.,0.,-1.));
#20289=DIRECTION('center_axis',(0.,0.,1.));
#20290=DIRECTION('ref_axis',(1.,0.,0.));
#20291=DIRECTION('center_axis',(0.,0.,1.));
#20292=DIRECTION('ref_axis',(1.,0.,0.));
#20293=DIRECTION('center_axis',(0.,0.,-1.));
#20294=DIRECTION('ref_axis',(1.,0.,0.));
#20295=DIRECTION('',(0.,0.,1.));
#20296=DIRECTION('center_axis',(0.,0.,1.));
#20297=DIRECTION('ref_axis',(1.,0.,0.));
#20298=DIRECTION('center_axis',(0.,0.,1.));
#20299=DIRECTION('ref_axis',(1.,0.,0.));
#20300=DIRECTION('',(0.64278760968653,0.766044443118986,0.));
#20301=DIRECTION('',(0.984807753012206,0.17364817766694,0.));
#20302=DIRECTION('',(-0.17364817766694,0.984807753012206,0.));
#20303=DIRECTION('',(0.984807753012206,0.17364817766694,0.));
#20304=DIRECTION('',(0.866025403784443,-0.499999999999992,0.));
#20305=DIRECTION('',(0.499999999999992,0.866025403784443,0.));
#20306=DIRECTION('',(0.866025403784443,-0.499999999999992,0.));
#20307=DIRECTION('',(0.342020143325676,-0.939692620785906,0.));
#20308=DIRECTION('',(0.939692620785906,0.342020143325676,0.));
#20309=DIRECTION('',(0.342020143325676,-0.939692620785906,0.));
#20310=DIRECTION('',(-0.342020143325663,-0.93969262078591,0.));
#20311=DIRECTION('',(0.93969262078591,-0.342020143325663,0.));
#20312=DIRECTION('',(-0.342020143325663,-0.93969262078591,0.));
#20313=DIRECTION('',(-0.866025403784436,-0.500000000000004,0.));
#20314=DIRECTION('',(0.500000000000004,-0.866025403784436,0.));
#20315=DIRECTION('',(-0.866025403784436,-0.500000000000004,0.));
#20316=DIRECTION('',(-0.984807753012209,0.173648177666927,0.));
#20317=DIRECTION('',(-0.173648177666927,-0.984807753012209,0.));
#20318=DIRECTION('',(-0.984807753012209,0.173648177666927,0.));
#20319=DIRECTION('',(-0.64278760968654,0.766044443118977,0.));
#20320=DIRECTION('',(-0.766044443118977,-0.64278760968654,0.));
#20321=DIRECTION('',(-0.64278760968654,0.766044443118977,0.));
#20322=DIRECTION('',(0.,1.,0.));
#20323=DIRECTION('',(-1.,0.,0.));
#20324=DIRECTION('',(0.,1.,0.));
#20325=DIRECTION('',(0.64278760968653,0.766044443118986,0.));
#20326=DIRECTION('',(-0.766044443118986,0.64278760968653,0.));
#20327=DIRECTION('center_axis',(0.,0.,1.));
#20328=DIRECTION('ref_axis',(1.,0.,0.));
#20329=DIRECTION('center_axis',(0.,0.,1.));
#20330=DIRECTION('ref_axis',(1.,0.,0.));
#20331=DIRECTION('center_axis',(0.,0.,1.));
#20332=DIRECTION('ref_axis',(1.,0.,0.));
#20333=DIRECTION('center_axis',(1.,1.26189474349424E-16,0.));
#20334=DIRECTION('ref_axis',(-1.26189474349424E-16,1.,0.));
#20335=DIRECTION('center_axis',(1.,1.26189474349424E-16,0.));
#20336=DIRECTION('ref_axis',(-1.26189474349424E-16,1.,0.));
#20337=DIRECTION('',(-1.38777878078145E-15,1.,0.));
#20338=DIRECTION('center_axis',(1.,1.26189474349424E-16,0.));
#20339=DIRECTION('ref_axis',(1.26189474349424E-16,-1.,0.));
#20340=DIRECTION('',(0.,0.,1.));
#20341=DIRECTION('center_axis',(1.,1.26189474349424E-16,0.));
#20342=DIRECTION('ref_axis',(1.26189474349424E-16,-1.,0.));
#20343=DIRECTION('',(1.38777878078145E-15,-1.,0.));
#20344=DIRECTION('center_axis',(1.,1.26189474349424E-16,0.));
#20345=DIRECTION('ref_axis',(1.26189474349424E-16,-1.,0.));
#20346=DIRECTION('',(0.,0.,-1.));
#20347=DIRECTION('center_axis',(1.,1.26189474349424E-16,0.));
#20348=DIRECTION('ref_axis',(-1.26189474349424E-16,1.,0.));
#20349=DIRECTION('center_axis',(1.,1.26189474349424E-16,0.));
#20350=DIRECTION('ref_axis',(-1.26189474349424E-16,1.,0.));
#20351=DIRECTION('',(0.,0.,-1.));
#20352=DIRECTION('center_axis',(1.,1.26189474349424E-16,0.));
#20353=DIRECTION('ref_axis',(1.26189474349424E-16,-1.,0.));
#20354=DIRECTION('',(1.38777878078145E-15,-1.,0.));
#20355=DIRECTION('center_axis',(1.,1.26189474349424E-16,0.));
#20356=DIRECTION('ref_axis',(1.26189474349424E-16,-1.,0.));
#20357=DIRECTION('',(0.,0.,1.));
#20358=DIRECTION('center_axis',(1.,1.26189474349424E-16,0.));
#20359=DIRECTION('ref_axis',(1.26189474349424E-16,-1.,0.));
#20360=DIRECTION('',(-1.38777878078145E-15,1.,0.));
#20361=DIRECTION('center_axis',(-1.,-1.26189474349424E-16,0.));
#20362=DIRECTION('ref_axis',(1.26189474349424E-16,-1.,0.));
#20363=DIRECTION('',(-1.,-1.26189474349424E-16,0.));
#20364=DIRECTION('',(-1.,-1.26189474349424E-16,0.));
#20365=DIRECTION('center_axis',(0.,0.,1.));
#20366=DIRECTION('ref_axis',(1.,0.,0.));
#20367=DIRECTION('',(-1.,-1.26189474349424E-16,0.));
#20368=DIRECTION('center_axis',(-1.,-1.26189474349424E-16,0.));
#20369=DIRECTION('ref_axis',(1.26189474349424E-16,-1.,0.));
#20370=DIRECTION('',(-1.,-1.26189474349424E-16,0.));
#20371=DIRECTION('center_axis',(1.26189474349424E-16,-1.,0.));
#20372=DIRECTION('ref_axis',(1.,1.26189474349424E-16,0.));
#20373=DIRECTION('',(-1.,-1.26189474349424E-16,0.));
#20374=DIRECTION('center_axis',(-1.,-1.26189474349424E-16,0.));
#20375=DIRECTION('ref_axis',(1.26189474349424E-16,-1.,0.));
#20376=DIRECTION('',(-1.,-1.26189474349424E-16,0.));
#20377=DIRECTION('center_axis',(0.,0.,-1.));
#20378=DIRECTION('ref_axis',(-1.,0.,0.));
#20379=DIRECTION('',(-1.,-1.26189474349424E-16,0.));
#20380=DIRECTION('center_axis',(-1.,-1.26189474349424E-16,0.));
#20381=DIRECTION('ref_axis',(1.26189474349424E-16,-1.,0.));
#20382=DIRECTION('',(-1.,-1.26189474349424E-16,0.));
#20383=DIRECTION('center_axis',(-1.26189474349424E-16,1.,0.));
#20384=DIRECTION('ref_axis',(-1.,-1.26189474349424E-16,0.));
#20385=DIRECTION('center_axis',(1.,1.26189474349424E-16,0.));
#20386=DIRECTION('ref_axis',(-1.26189474349424E-16,1.,0.));
#20387=DIRECTION('center_axis',(1.,1.26189474349424E-16,0.));
#20388=DIRECTION('ref_axis',(-1.26189474349424E-16,1.,0.));
#20389=DIRECTION('',(-1.38777878078145E-15,1.,0.));
#20390=DIRECTION('center_axis',(1.,1.26189474349424E-16,0.));
#20391=DIRECTION('ref_axis',(1.26189474349424E-16,-1.,0.));
#20392=DIRECTION('',(0.,0.,1.));
#20393=DIRECTION('center_axis',(1.,1.26189474349424E-16,0.));
#20394=DIRECTION('ref_axis',(-1.26189474349424E-16,1.,0.));
#20395=DIRECTION('',(1.38777878078145E-15,-1.,0.));
#20396=DIRECTION('center_axis',(1.,1.26189474349424E-16,0.));
#20397=DIRECTION('ref_axis',(-1.26189474349424E-16,1.,0.));
#20398=DIRECTION('',(0.,0.,-1.));
#20399=DIRECTION('center_axis',(1.,1.26189474349424E-16,0.));
#20400=DIRECTION('ref_axis',(-1.26189474349424E-16,1.,0.));
#20401=DIRECTION('center_axis',(1.,1.26189474349424E-16,0.));
#20402=DIRECTION('ref_axis',(-1.26189474349424E-16,1.,0.));
#20403=DIRECTION('',(0.,0.,-1.));
#20404=DIRECTION('center_axis',(1.,1.26189474349424E-16,0.));
#20405=DIRECTION('ref_axis',(-1.26189474349424E-16,1.,0.));
#20406=DIRECTION('',(1.38777878078145E-15,-1.,0.));
#20407=DIRECTION('center_axis',(1.,1.26189474349424E-16,0.));
#20408=DIRECTION('ref_axis',(-1.26189474349424E-16,1.,0.));
#20409=DIRECTION('',(0.,0.,1.));
#20410=DIRECTION('center_axis',(1.,1.26189474349424E-16,0.));
#20411=DIRECTION('ref_axis',(1.26189474349424E-16,-1.,0.));
#20412=DIRECTION('',(-1.38777878078145E-15,1.,0.));
#20413=DIRECTION('center_axis',(-1.,-1.26189474349424E-16,0.));
#20414=DIRECTION('ref_axis',(1.26189474349424E-16,-1.,0.));
#20415=DIRECTION('',(-1.,-1.26189474349424E-16,0.));
#20416=DIRECTION('',(-1.,-1.26189474349424E-16,0.));
#20417=DIRECTION('center_axis',(0.,0.,1.));
#20418=DIRECTION('ref_axis',(1.,0.,0.));
#20419=DIRECTION('',(-1.,-1.26189474349424E-16,0.));
#20420=DIRECTION('center_axis',(-1.,-1.26189474349424E-16,0.));
#20421=DIRECTION('ref_axis',(1.26189474349424E-16,-1.,0.));
#20422=DIRECTION('',(-1.,-1.26189474349424E-16,0.));
#20423=DIRECTION('center_axis',(1.26189474349424E-16,-1.,0.));
#20424=DIRECTION('ref_axis',(1.,1.26189474349424E-16,0.));
#20425=DIRECTION('',(-1.,-1.26189474349424E-16,0.));
#20426=DIRECTION('center_axis',(-1.,-1.26189474349424E-16,0.));
#20427=DIRECTION('ref_axis',(1.26189474349424E-16,-1.,0.));
#20428=DIRECTION('',(-1.,-1.26189474349424E-16,0.));
#20429=DIRECTION('center_axis',(0.,0.,-1.));
#20430=DIRECTION('ref_axis',(-1.,0.,0.));
#20431=DIRECTION('',(-1.,-1.26189474349424E-16,0.));
#20432=DIRECTION('center_axis',(-1.,-1.26189474349424E-16,0.));
#20433=DIRECTION('ref_axis',(1.26189474349424E-16,-1.,0.));
#20434=DIRECTION('',(-1.,-1.26189474349424E-16,0.));
#20435=DIRECTION('center_axis',(-1.26189474349424E-16,1.,0.));
#20436=DIRECTION('ref_axis',(-1.,-1.26189474349424E-16,0.));
#20437=DIRECTION('center_axis',(0.,0.,1.));
#20438=DIRECTION('ref_axis',(1.,0.,0.));
#20439=DIRECTION('center_axis',(1.,0.,0.));
#20440=DIRECTION('ref_axis',(0.,0.,-1.));
#20441=DIRECTION('',(0.,-0.955520783784934,0.294923772787182));
#20442=DIRECTION('center_axis',(1.,0.,0.));
#20443=DIRECTION('ref_axis',(0.,0.,-1.));
#20444=DIRECTION('',(0.,-0.955520783784934,0.294923772787182));
#20445=DIRECTION('center_axis',(0.,-0.294923772787182,-0.955520783784934));
#20446=DIRECTION('ref_axis',(0.,0.955520783784934,-0.294923772787182));
#20447=DIRECTION('center_axis',(0.766044443118977,0.64278760968654,0.));
#20448=DIRECTION('ref_axis',(0.,0.,-1.));
#20449=DIRECTION('',(0.614196920614927,-0.731971386703138,0.294923772787182));
#20450=DIRECTION('center_axis',(0.766044443118977,0.64278760968654,0.));
#20451=DIRECTION('ref_axis',(0.,0.,-1.));
#20452=DIRECTION('',(0.614196920614927,-0.731971386703138,0.294923772787182));
#20453=DIRECTION('center_axis',(0.189573346949609,-0.225924717287304,-0.955520783784934));
#20454=DIRECTION('ref_axis',(5.1741255323139E-18,0.973167658917659,-0.230097169988514));
#20455=DIRECTION('center_axis',(0.173648177666927,0.984807753012209,0.));
#20456=DIRECTION('ref_axis',(0.,0.,-1.));
#20457=DIRECTION('',(0.941004276035705,-0.165924442827128,0.294923772787182));
#20458=DIRECTION('center_axis',(0.173648177666927,0.984807753012209,0.));
#20459=DIRECTION('ref_axis',(0.,0.,-1.));
#20460=DIRECTION('',(0.941004276035705,-0.165924442827128,0.294923772787182));
#20461=DIRECTION('center_axis',(0.290443217988428,-0.0512129756951491,-0.955520783784934));
#20462=DIRECTION('ref_axis',(-0.95677630912777,-2.49539129740611E-18,-0.290824851571943));
#20463=DIRECTION('center_axis',(-0.500000000000004,0.866025403784436,0.));
#20464=DIRECTION('ref_axis',(0.,0.,-1.));
#20465=DIRECTION('',(0.827505272601769,0.477760391892471,0.294923772787182));
#20466=DIRECTION('center_axis',(-0.500000000000004,0.866025403784436,0.));
#20467=DIRECTION('ref_axis',(0.,0.,-1.));
#20468=DIRECTION('',(0.827505272601769,0.477760391892471,0.294923772787182));
#20469=DIRECTION('center_axis',(0.255411479413649,0.147461886393592,-0.955520783784934));
#20470=DIRECTION('ref_axis',(-0.966082247190219,-2.695277852006E-19,-0.25823456713596));
#20471=DIRECTION('center_axis',(-0.939692620785911,0.342020143325663,0.));
#20472=DIRECTION('ref_axis',(0.,0.,-1.));
#20473=DIRECTION('',(0.326807355420773,0.897895829530272,0.294923772787182));
#20474=DIRECTION('center_axis',(-0.939692620785911,0.342020143325663,0.));
#20475=DIRECTION('ref_axis',(0.,0.,-1.));
#20476=DIRECTION('',(0.326807355420773,0.897895829530272,0.294923772787182));
#20477=DIRECTION('center_axis',(0.100869871038817,0.277137692982455,-0.955520783784934));
#20478=DIRECTION('ref_axis',(2.8977398537934E-18,0.960419279714667,0.278558444769426));
#20479=DIRECTION('center_axis',(-0.939692620785906,-0.342020143325676,0.));
#20480=DIRECTION('ref_axis',(0.,0.,-1.));
#20481=DIRECTION('',(-0.326807355420785,0.897895829530268,0.294923772787182));
#20482=DIRECTION('center_axis',(-0.939692620785906,-0.342020143325676,0.));
#20483=DIRECTION('ref_axis',(0.,0.,-1.));
#20484=DIRECTION('',(-0.326807355420785,0.897895829530268,0.294923772787182));
#20485=DIRECTION('center_axis',(-0.100869871038821,0.277137692982454,-0.955520783784934));
#20486=DIRECTION('ref_axis',(-1.67311827781928E-19,0.960419279714667,0.278558444769425));
#20487=DIRECTION('center_axis',(-0.499999999999992,-0.866025403784443,0.));
#20488=DIRECTION('ref_axis',(0.,0.,-1.));
#20489=DIRECTION('',(-0.827505272601775,0.477760391892459,0.294923772787182));
#20490=DIRECTION('center_axis',(-0.499999999999992,-0.866025403784443,0.));
#20491=DIRECTION('ref_axis',(0.,0.,-1.));
#20492=DIRECTION('',(-0.827505272601775,0.477760391892459,0.294923772787182));
#20493=DIRECTION('center_axis',(-0.255411479413651,0.147461886393589,-0.955520783784934));
#20494=DIRECTION('ref_axis',(-0.966082247190218,-1.82035480917452E-18,0.258234567135962));
#20495=DIRECTION('center_axis',(0.17364817766694,-0.984807753012206,0.));
#20496=DIRECTION('ref_axis',(0.,0.,-1.));
#20497=DIRECTION('',(-0.941004276035703,-0.16592444282714,0.294923772787182));
#20498=DIRECTION('center_axis',(0.17364817766694,-0.984807753012206,0.));
#20499=DIRECTION('ref_axis',(0.,0.,-1.));
#20500=DIRECTION('',(-0.941004276035703,-0.16592444282714,0.294923772787182));
#20501=DIRECTION('center_axis',(-0.290443217988427,-0.0512129756951529,
-0.955520783784934));
#20502=DIRECTION('ref_axis',(-0.95677630912777,-5.00082995194373E-19,0.290824851571942));
#20503=DIRECTION('center_axis',(0.766044443118986,-0.64278760968653,0.));
#20504=DIRECTION('ref_axis',(0.,0.,-1.));
#20505=DIRECTION('',(-0.614196920614917,-0.731971386703147,0.294923772787182));
#20506=DIRECTION('center_axis',(0.766044443118986,-0.64278760968653,0.));
#20507=DIRECTION('ref_axis',(0.,0.,-1.));
#20508=DIRECTION('',(-0.614196920614917,-0.731971386703147,0.294923772787182));
#20509=DIRECTION('center_axis',(-0.189573346949606,-0.225924717287307,-0.955520783784934));
#20510=DIRECTION('ref_axis',(4.39360789729016E-18,0.973167658917658,-0.230097169988516));
#24906=CARTESIAN_POINT('',(0.,0.,0.));
#24907=CARTESIAN_POINT('Origin',(0.,0.,-50.));
#24908=CARTESIAN_POINT('',(-30.,-3.67394039744206E-15,-55.));
#24909=CARTESIAN_POINT('Origin',(0.,0.,-55.));
#24910=CARTESIAN_POINT('',(-25.,-3.06161699786838E-15,-50.));
#24911=CARTESIAN_POINT('Origin',(-30.,-3.67394039744206E-15,-50.));
#24912=CARTESIAN_POINT('Origin',(0.,0.,-50.));
#24913=CARTESIAN_POINT('Origin',(0.,0.,-50.));
#24914=CARTESIAN_POINT('',(250.,3.06161699786838E-14,-50.));
#24915=CARTESIAN_POINT('',(-250.,-3.06161699786838E-14,-50.));
#24916=CARTESIAN_POINT('Origin',(0.,0.,-50.));
#24917=CARTESIAN_POINT('Origin',(0.,0.,-50.));
#24918=CARTESIAN_POINT('',(-245.,-3.00038465791102E-14,-55.));
#24919=CARTESIAN_POINT('Origin',(-245.,-3.00038465791102E-14,-50.));
#24920=CARTESIAN_POINT('Origin',(0.,0.,-55.));
#24921=CARTESIAN_POINT('Origin',(0.,0.,-35.));
#24922=CARTESIAN_POINT('',(-34.8143500942353,3.60014270772951,-45.));
#24923=CARTESIAN_POINT('',(-31.4834665561195,-15.2902365452502,-45.));
#24924=CARTESIAN_POINT('Origin',(0.,0.,-45.));
#24925=CARTESIAN_POINT('',(-31.4834665561195,-15.2902365452502,-36.5156684558794));
#24926=CARTESIAN_POINT('',(-31.4834665561195,-15.2902365452502,-35.));
#24927=CARTESIAN_POINT('',(-28.9834665561195,-19.6203635641724,-36.5156684558794));
#24928=CARTESIAN_POINT('Origin',(0.,0.,-25.7404283258302));
#24929=CARTESIAN_POINT('',(-28.9834665561195,-19.6203635641724,-45.));
#24930=CARTESIAN_POINT('',(-28.9834665561195,-19.6203635641724,-35.));
#24931=CARTESIAN_POINT('',(-14.2893600049743,-31.9501829517178,-45.));
#24932=CARTESIAN_POINT('Origin',(0.,0.,-45.));
#24933=CARTESIAN_POINT('',(-14.2893600049743,-31.9501829517178,-36.5156684558794));
#24934=CARTESIAN_POINT('',(-14.2893600049743,-31.9501829517178,-35.));
#24935=CARTESIAN_POINT('',(-9.59089690104477,-33.6602836683462,-36.5156684558794));
#24936=CARTESIAN_POINT('Origin',(0.,0.,-25.7404283258302));
#24937=CARTESIAN_POINT('',(-9.59089690104477,-33.6602836683461,-45.));
#24938=CARTESIAN_POINT('',(-9.59089690104477,-33.6602836683462,-35.));
#24939=CARTESIAN_POINT('',(9.59089690104522,-33.660283668346,-45.));
#24940=CARTESIAN_POINT('Origin',(0.,0.,-45.));
#24941=CARTESIAN_POINT('',(9.59089690104522,-33.660283668346,-36.5156684558794));
#24942=CARTESIAN_POINT('',(9.59089690104522,-33.660283668346,-35.));
#24943=CARTESIAN_POINT('',(14.2893600049748,-31.9501829517176,-36.5156684558794));
#24944=CARTESIAN_POINT('Origin',(0.,0.,-25.7404283258302));
#24945=CARTESIAN_POINT('',(14.2893600049748,-31.9501829517176,-45.));
#24946=CARTESIAN_POINT('',(14.2893600049748,-31.9501829517176,-35.));
#24947=CARTESIAN_POINT('',(28.9834665561198,-19.620363564172,-45.));
#24948=CARTESIAN_POINT('Origin',(0.,0.,-45.));
#24949=CARTESIAN_POINT('',(28.9834665561198,-19.620363564172,-36.5156684558794));
#24950=CARTESIAN_POINT('',(28.9834665561198,-19.620363564172,-35.));
#24951=CARTESIAN_POINT('',(31.4834665561197,-15.2902365452498,-36.5156684558794));
#24952=CARTESIAN_POINT('Origin',(0.,0.,-25.7404283258302));
#24953=CARTESIAN_POINT('',(31.4834665561197,-15.2902365452498,-45.));
#24954=CARTESIAN_POINT('',(31.4834665561197,-15.2902365452498,-35.));
#24955=CARTESIAN_POINT('',(35.,-4.28626379701574E-15,-45.));
#24956=CARTESIAN_POINT('Origin',(0.,0.,-45.));
#24957=CARTESIAN_POINT('',(35.,-4.28626379701574E-15,-35.));
#24958=CARTESIAN_POINT('',(35.,-4.28626379701574E-15,-35.));
#24959=CARTESIAN_POINT('Origin',(0.,0.,-35.));
#24960=CARTESIAN_POINT('',(34.8143500942353,3.60014270772997,-45.));
#24961=CARTESIAN_POINT('Origin',(0.,0.,-45.));
#24962=CARTESIAN_POINT('',(34.8143500942353,3.60014270772997,-36.5156684558794));
#24963=CARTESIAN_POINT('',(34.8143500942353,3.60014270772997,-35.));
#24964=CARTESIAN_POINT('',(33.9461092059006,8.524181472791,-36.5156684558794));
#24965=CARTESIAN_POINT('Origin',(0.,0.,-25.7404283258302));
#24966=CARTESIAN_POINT('',(33.9461092059006,8.524181472791,-45.));
#24967=CARTESIAN_POINT('',(33.9461092059006,8.524181472791,-35.));
#24968=CARTESIAN_POINT('',(24.3552123048554,25.1361021955557,-45.));
#24969=CARTESIAN_POINT('Origin',(0.,0.,-45.));
#24970=CARTESIAN_POINT('',(24.3552123048554,25.1361021955557,-36.5156684558794));
#24971=CARTESIAN_POINT('',(24.3552123048554,25.1361021955557,-35.));
#24972=CARTESIAN_POINT('',(20.5249900892604,28.3500402439884,-36.5156684558794));
#24973=CARTESIAN_POINT('Origin',(0.,0.,-25.7404283258302));
#24974=CARTESIAN_POINT('',(20.5249900892604,28.3500402439884,-45.));
#24975=CARTESIAN_POINT('',(20.5249900892604,28.3500402439884,-35.));
#24976=CARTESIAN_POINT('',(2.5,34.9106001094224,-45.));
#24977=CARTESIAN_POINT('Origin',(0.,0.,-45.));
#24978=CARTESIAN_POINT('',(2.5,34.9106001094224,-36.5156684558794));
#24979=CARTESIAN_POINT('',(2.5,34.9106001094224,-35.));
#24980=CARTESIAN_POINT('',(-2.5,34.9106001094224,-36.5156684558794));
#24981=CARTESIAN_POINT('Origin',(0.,0.,-25.7404283258302));
#24982=CARTESIAN_POINT('',(-2.5,34.9106001094224,-45.));
#24983=CARTESIAN_POINT('',(-2.5,34.9106001094224,-35.));
#24984=CARTESIAN_POINT('',(-20.5249900892608,28.3500402439881,-45.));
#24985=CARTESIAN_POINT('Origin',(0.,0.,-45.));
#24986=CARTESIAN_POINT('',(-20.5249900892608,28.3500402439881,-36.5156684558794));
#24987=CARTESIAN_POINT('',(-20.5249900892608,28.3500402439881,-35.));
#24988=CARTESIAN_POINT('',(-24.3552123048557,25.1361021955554,-36.5156684558794));
#24989=CARTESIAN_POINT('Origin',(0.,0.,-25.7404283258302));
#24990=CARTESIAN_POINT('',(-24.3552123048557,25.1361021955554,-45.));
#24991=CARTESIAN_POINT('',(-24.3552123048557,25.1361021955554,-35.));
#24992=CARTESIAN_POINT('',(-33.9461092059007,8.52418147279055,-45.));
#24993=CARTESIAN_POINT('Origin',(0.,0.,-45.));
#24994=CARTESIAN_POINT('',(-33.9461092059007,8.52418147279055,-36.5156684558794));
#24995=CARTESIAN_POINT('',(-33.9461092059007,8.52418147279055,-35.));
#24996=CARTESIAN_POINT('',(-34.8143500942353,3.60014270772951,-36.5156684558794));
#24997=CARTESIAN_POINT('Origin',(0.,0.,-25.7404283258302));
#24998=CARTESIAN_POINT('',(-34.8143500942353,3.60014270772951,-35.));
#24999=CARTESIAN_POINT('Origin',(263.115760998171,-242.,-20.));
#25000=CARTESIAN_POINT('',(263.115760998171,-239.5,-20.));
#25001=CARTESIAN_POINT('Origin',(263.115760998171,-242.,-20.));
#25002=CARTESIAN_POINT('',(258.115760998171,-239.5,-20.));
#25003=CARTESIAN_POINT('',(263.115760998171,-239.5,-20.));
#25004=CARTESIAN_POINT('Origin',(258.115760998171,-242.,-20.));
#25005=CARTESIAN_POINT('Origin',(263.115760998171,-242.,20.));
#25006=CARTESIAN_POINT('',(263.115760998171,-239.5,20.));
#25007=CARTESIAN_POINT('Origin',(263.115760998171,-242.,20.));
#25008=CARTESIAN_POINT('',(258.115760998171,-239.5,20.));
#25009=CARTESIAN_POINT('',(263.115760998171,-239.5,20.));
#25010=CARTESIAN_POINT('Origin',(258.115760998171,-242.,20.));
#25011=CARTESIAN_POINT('Origin',(263.115760998171,-202.,20.));
#25012=CARTESIAN_POINT('',(263.115760998171,-199.5,20.));
#25013=CARTESIAN_POINT('Origin',(263.115760998171,-202.,20.));
#25014=CARTESIAN_POINT('',(258.115760998171,-199.5,20.));
#25015=CARTESIAN_POINT('',(263.115760998171,-199.5,20.));
#25016=CARTESIAN_POINT('Origin',(258.115760998171,-202.,20.));
#25017=CARTESIAN_POINT('Origin',(263.115760998171,-202.,-20.));
#25018=CARTESIAN_POINT('',(263.115760998171,-199.5,-20.));
#25019=CARTESIAN_POINT('Origin',(263.115760998171,-202.,-20.));
#25020=CARTESIAN_POINT('',(258.115760998171,-199.5,-20.));
#25021=CARTESIAN_POINT('',(263.115760998171,-199.5,-20.));
#25022=CARTESIAN_POINT('Origin',(258.115760998171,-202.,-20.));
#25023=CARTESIAN_POINT('Origin',(263.11576099817,242.,20.));
#25024=CARTESIAN_POINT('',(263.11576099817,244.5,20.));
#25025=CARTESIAN_POINT('Origin',(263.11576099817,242.,20.));
#25026=CARTESIAN_POINT('',(258.11576099817,244.5,20.));
#25027=CARTESIAN_POINT('',(263.11576099817,244.5,20.));
#25028=CARTESIAN_POINT('Origin',(258.11576099817,242.,20.));
#25029=CARTESIAN_POINT('Origin',(263.115760998171,202.,-20.));
#25030=CARTESIAN_POINT('',(263.115760998171,204.5,-20.));
#25031=CARTESIAN_POINT('Origin',(263.115760998171,202.,-20.));
#25032=CARTESIAN_POINT('',(258.115760998171,204.5,-20.));
#25033=CARTESIAN_POINT('',(263.115760998171,204.5,-20.));
#25034=CARTESIAN_POINT('Origin',(258.115760998171,202.,-20.));
#25035=CARTESIAN_POINT('Origin',(263.115760998171,202.,20.));
#25036=CARTESIAN_POINT('',(263.115760998171,204.5,20.));
#25037=CARTESIAN_POINT('Origin',(263.115760998171,202.,20.));
#25038=CARTESIAN_POINT('',(258.115760998171,204.5,20.));
#25039=CARTESIAN_POINT('',(263.115760998171,204.5,20.));
#25040=CARTESIAN_POINT('Origin',(258.115760998171,202.,20.));
#25041=CARTESIAN_POINT('Origin',(263.11576099817,242.,-20.));
#25042=CARTESIAN_POINT('',(263.11576099817,244.5,-20.));
#25043=CARTESIAN_POINT('Origin',(263.11576099817,242.,-20.));
#25044=CARTESIAN_POINT('',(258.11576099817,244.5,-20.));
#25045=CARTESIAN_POINT('',(263.11576099817,244.5,-20.));
#25046=CARTESIAN_POINT('Origin',(258.11576099817,242.,-20.));
#25047=CARTESIAN_POINT('Origin',(258.11576099817,222.,0.));
#25048=CARTESIAN_POINT('',(66.475559418481,241.,2.32682891837986E-15));
#25049=CARTESIAN_POINT('Ctrl Pts',(66.475559418481,241.,6.03683769639929E-15));
#25050=CARTESIAN_POINT('Ctrl Pts',(66.475559418481,241.,-0.818914397616676));
#25051=CARTESIAN_POINT('Ctrl Pts',(66.6828156889532,240.943036471407,-1.66914044272295));
#25052=CARTESIAN_POINT('Ctrl Pts',(67.4158253648335,240.738969075332,-3.23661719250768));
#25053=CARTESIAN_POINT('Ctrl Pts',(67.933482619513,240.59373120234,-3.95788330423287));
#25054=CARTESIAN_POINT('Ctrl Pts',(69.6361378266225,240.108932801212,-5.91638068595454));
#25055=CARTESIAN_POINT('Ctrl Pts',(71.1576540050022,239.665242818586,-7.08907003196721));
#25056=CARTESIAN_POINT('Ctrl Pts',(74.3823681679428,238.684108540751,-9.16276251679134));
#25057=CARTESIAN_POINT('Ctrl Pts',(76.0892097916356,238.145315558933,-10.0574548511805));
#25058=CARTESIAN_POINT('Ctrl Pts',(80.5078069493414,236.701116337081,-12.1466632640978));
#25059=CARTESIAN_POINT('Ctrl Pts',(83.5441791540702,235.651195580973,-13.3041009898948));
#25060=CARTESIAN_POINT('Ctrl Pts',(89.798722524918,233.339463641051,-15.32223219563));
#25061=CARTESIAN_POINT('Ctrl Pts',(93.0181628755071,232.0771819994,-16.1784506413274));
#25062=CARTESIAN_POINT('Ctrl Pts',(99.4647393270101,229.388236379592,-17.5700183736559));
#25063=CARTESIAN_POINT('Ctrl Pts',(102.691654775973,227.961595935903,-18.1038606242188));
#25064=CARTESIAN_POINT('Ctrl Pts',(108.98538364367,225.020557582189,-18.8193152708395));
#25065=CARTESIAN_POINT('Ctrl Pts',(112.052307853074,223.506171165075,-19.));
#25066=CARTESIAN_POINT('Ctrl Pts',(119.299384453378,219.753332518616,-19.));
#25067=CARTESIAN_POINT('Ctrl Pts',(123.97020433053,217.157824280152,-18.593013611366));
#25068=CARTESIAN_POINT('Ctrl Pts',(130.550318589395,213.220888597628,-16.9104681529982));
#25069=CARTESIAN_POINT('Ctrl Pts',(132.673701403444,211.903864145767,-16.1734222030093));
#25070=CARTESIAN_POINT('Ctrl Pts',(136.64657075335,209.363973465165,-14.2773379372075));
#25071=CARTESIAN_POINT('Ctrl Pts',(138.497260071169,208.140453793306,-13.1216968983942));
#25072=CARTESIAN_POINT('Ctrl Pts',(140.914378515077,206.504262153928,-11.0274797072174));
#25073=CARTESIAN_POINT('Ctrl Pts',(141.679048846267,205.980033579842,-10.2626502639426));
#25074=CARTESIAN_POINT('Ctrl Pts',(143.080866831829,205.008762402486,-8.55915648524146));
#25075=CARTESIAN_POINT('Ctrl Pts',(143.717851327755,204.561968106359,-7.62021633376244));
#25076=CARTESIAN_POINT('Ctrl Pts',(144.775897909994,203.814520750128,-5.60723443384186));
#25077=CARTESIAN_POINT('Ctrl Pts',(145.197945099354,203.513339264161,-4.53064652501085));
#25078=CARTESIAN_POINT('Ctrl Pts',(145.767257174916,203.105955734851,-2.30184157443626));
#25079=CARTESIAN_POINT('Ctrl Pts',(145.914358443575,203.,-1.14953772934859));
#25080=CARTESIAN_POINT('Ctrl Pts',(145.914358443575,203.,1.14953772934859));
#25081=CARTESIAN_POINT('Ctrl Pts',(145.767257174916,203.105955734851,2.30184157443626));
#25082=CARTESIAN_POINT('Ctrl Pts',(145.197945099354,203.513339264161,4.53064652501085));
#25083=CARTESIAN_POINT('Ctrl Pts',(144.775897909994,203.814520750128,5.60723443384185));
#25084=CARTESIAN_POINT('Ctrl Pts',(143.717851327755,204.561968106359,7.62021633376245));
#25085=CARTESIAN_POINT('Ctrl Pts',(143.080866831829,205.008762402486,8.55915648524148));
#25086=CARTESIAN_POINT('Ctrl Pts',(141.679048846267,205.980033579842,10.2626502639426));
#25087=CARTESIAN_POINT('Ctrl Pts',(140.914378515077,206.504262153928,11.0274797072174));
#25088=CARTESIAN_POINT('Ctrl Pts',(138.497260071169,208.140453793306,13.1216968983942));
#25089=CARTESIAN_POINT('Ctrl Pts',(136.64657075335,209.363973465165,14.2773379372075));
#25090=CARTESIAN_POINT('Ctrl Pts',(132.673701403444,211.903864145767,16.1734222030093));
#25091=CARTESIAN_POINT('Ctrl Pts',(130.550318589395,213.220888597628,16.9104681529982));
#25092=CARTESIAN_POINT('Ctrl Pts',(123.97020433053,217.157824280152,18.593013611366));
#25093=CARTESIAN_POINT('Ctrl Pts',(119.299384453378,219.753332518616,19.));
#25094=CARTESIAN_POINT('Ctrl Pts',(112.052307853074,223.506171165075,19.));
#25095=CARTESIAN_POINT('Ctrl Pts',(108.98538364367,225.020557582189,18.8193152708395));
#25096=CARTESIAN_POINT('Ctrl Pts',(102.691654775973,227.961595935903,18.1038606242188));
#25097=CARTESIAN_POINT('Ctrl Pts',(99.4647393270101,229.388236379592,17.5700183736559));
#25098=CARTESIAN_POINT('Ctrl Pts',(93.0181628755072,232.0771819994,16.1784506413274));
#25099=CARTESIAN_POINT('Ctrl Pts',(89.798722524918,233.339463641051,15.32223219563));
#25100=CARTESIAN_POINT('Ctrl Pts',(83.5441791540702,235.651195580973,13.3041009898948));
#25101=CARTESIAN_POINT('Ctrl Pts',(80.5078069493414,236.701116337081,12.1466632640978));
#25102=CARTESIAN_POINT('Ctrl Pts',(76.0892097916356,238.145315558933,10.0574548511805));
#25103=CARTESIAN_POINT('Ctrl Pts',(74.3823681679427,238.684108540751,9.16276251679135));
#25104=CARTESIAN_POINT('Ctrl Pts',(71.1576540050022,239.665242818586,7.08907003196723));
#25105=CARTESIAN_POINT('Ctrl Pts',(69.6361378266225,240.108932801212,5.91638068595453));
#25106=CARTESIAN_POINT('Ctrl Pts',(67.933482619513,240.59373120234,3.95788330423286));
#25107=CARTESIAN_POINT('Ctrl Pts',(67.4158253648334,240.738969075332,3.23661719250768));
#25108=CARTESIAN_POINT('Ctrl Pts',(66.6828156889532,240.943036471406,1.66914044272293));
#25109=CARTESIAN_POINT('Ctrl Pts',(66.475559418481,241.,0.818914397616675));
#25110=CARTESIAN_POINT('Ctrl Pts',(66.475559418481,241.,-8.32667268468867E-16));
#25111=CARTESIAN_POINT('',(258.11576099817,241.,-2.32682891837997E-15));
#25112=CARTESIAN_POINT('',(258.11576099817,241.,-2.32682891837997E-15));
#25113=CARTESIAN_POINT('Origin',(258.11576099817,222.,0.));
#25114=CARTESIAN_POINT('Origin',(258.115760998171,-222.,0.));
#25115=CARTESIAN_POINT('',(145.914358443575,-203.,0.));
#25116=CARTESIAN_POINT('Ctrl Pts',(145.914358443575,-203.,1.94289029309402E-15));
#25117=CARTESIAN_POINT('Ctrl Pts',(145.914358443575,-203.,-1.14953772934859));
#25118=CARTESIAN_POINT('Ctrl Pts',(145.767257174916,-203.105955734851,-2.30184157443626));
#25119=CARTESIAN_POINT('Ctrl Pts',(145.197945099354,-203.513339264161,-4.53064652501085));
#25120=CARTESIAN_POINT('Ctrl Pts',(144.775897909994,-203.814520750128,-5.60723443384187));
#25121=CARTESIAN_POINT('Ctrl Pts',(143.717851327755,-204.561968106359,-7.62021633376246));
#25122=CARTESIAN_POINT('Ctrl Pts',(143.080866831829,-205.008762402486,-8.55915648524147));
#25123=CARTESIAN_POINT('Ctrl Pts',(141.679048846267,-205.980033579842,-10.2626502639426));
#25124=CARTESIAN_POINT('Ctrl Pts',(140.914378515077,-206.504262153928,-11.0274797072174));
#25125=CARTESIAN_POINT('Ctrl Pts',(138.497260071169,-208.140453793306,-13.1216968983942));
#25126=CARTESIAN_POINT('Ctrl Pts',(136.64657075335,-209.363973465165,-14.2773379372076));
#25127=CARTESIAN_POINT('Ctrl Pts',(132.673701403444,-211.903864145766,-16.1734222030094));
#25128=CARTESIAN_POINT('Ctrl Pts',(130.550318589395,-213.220888597628,-16.9104681529982));
#25129=CARTESIAN_POINT('Ctrl Pts',(123.97020433053,-217.157824280152,-18.593013611366));
#25130=CARTESIAN_POINT('Ctrl Pts',(119.299384453378,-219.753332518616,-19.));
#25131=CARTESIAN_POINT('Ctrl Pts',(112.052307853074,-223.506171165075,-19.));
#25132=CARTESIAN_POINT('Ctrl Pts',(108.98538364367,-225.020557582189,-18.8193152708395));
#25133=CARTESIAN_POINT('Ctrl Pts',(102.691654775973,-227.961595935903,-18.1038606242189));
#25134=CARTESIAN_POINT('Ctrl Pts',(99.46473932701,-229.388236379592,-17.570018373656));
#25135=CARTESIAN_POINT('Ctrl Pts',(93.0181628755071,-232.0771819994,-16.1784506413275));
#25136=CARTESIAN_POINT('Ctrl Pts',(89.7987225249179,-233.339463641051,-15.32223219563));
#25137=CARTESIAN_POINT('Ctrl Pts',(83.5441791540701,-235.651195580973,-13.3041009898948));
#25138=CARTESIAN_POINT('Ctrl Pts',(80.5078069493413,-236.701116337082,-12.1466632640978));
#25139=CARTESIAN_POINT('Ctrl Pts',(76.0892097916354,-238.145315558933,-10.0574548511805));
#25140=CARTESIAN_POINT('Ctrl Pts',(74.3823681679425,-238.684108540751,-9.16276251679143));
#25141=CARTESIAN_POINT('Ctrl Pts',(71.157654005002,-239.665242818586,-7.08907003196732));
#25142=CARTESIAN_POINT('Ctrl Pts',(69.6361378266224,-240.108932801212,-5.91638068595454));
#25143=CARTESIAN_POINT('Ctrl Pts',(67.9334826195128,-240.593731202341,-3.95788330423287));
#25144=CARTESIAN_POINT('Ctrl Pts',(67.4158253648332,-240.738969075332,-3.23661719250773));
#25145=CARTESIAN_POINT('Ctrl Pts',(66.6828156889529,-240.943036471407,-1.669140442723));
#25146=CARTESIAN_POINT('Ctrl Pts',(66.4755594184807,-241.,-0.818914397616677));
#25147=CARTESIAN_POINT('Ctrl Pts',(66.4755594184807,-241.,0.818914397616677));
#25148=CARTESIAN_POINT('Ctrl Pts',(66.6828156889529,-240.943036471407,1.669140442723));
#25149=CARTESIAN_POINT('Ctrl Pts',(67.4158253648332,-240.738969075332,3.23661719250773));
#25150=CARTESIAN_POINT('Ctrl Pts',(67.9334826195128,-240.593731202341,3.95788330423287));
#25151=CARTESIAN_POINT('Ctrl Pts',(69.6361378266224,-240.108932801212,5.91638068595454));
#25152=CARTESIAN_POINT('Ctrl Pts',(71.157654005002,-239.665242818586,7.0890700319673));
#25153=CARTESIAN_POINT('Ctrl Pts',(74.3823681679425,-238.684108540751,9.1627625167914));
#25154=CARTESIAN_POINT('Ctrl Pts',(76.0892097916354,-238.145315558933,10.0574548511805));
#25155=CARTESIAN_POINT('Ctrl Pts',(80.5078069493413,-236.701116337082,12.1466632640978));
#25156=CARTESIAN_POINT('Ctrl Pts',(83.5441791540701,-235.651195580973,13.3041009898948));
#25157=CARTESIAN_POINT('Ctrl Pts',(89.7987225249179,-233.339463641051,15.32223219563));
#25158=CARTESIAN_POINT('Ctrl Pts',(93.0181628755071,-232.0771819994,16.1784506413275));
#25159=CARTESIAN_POINT('Ctrl Pts',(99.46473932701,-229.388236379592,17.570018373656));
#25160=CARTESIAN_POINT('Ctrl Pts',(102.691654775973,-227.961595935903,18.1038606242189));
#25161=CARTESIAN_POINT('Ctrl Pts',(108.98538364367,-225.020557582189,18.8193152708395));
#25162=CARTESIAN_POINT('Ctrl Pts',(112.052307853074,-223.506171165075,19.));
#25163=CARTESIAN_POINT('Ctrl Pts',(119.299384453378,-219.753332518616,19.));
#25164=CARTESIAN_POINT('Ctrl Pts',(123.97020433053,-217.157824280152,18.593013611366));
#25165=CARTESIAN_POINT('Ctrl Pts',(130.550318589395,-213.220888597628,16.9104681529982));
#25166=CARTESIAN_POINT('Ctrl Pts',(132.673701403444,-211.903864145766,16.1734222030093));
#25167=CARTESIAN_POINT('Ctrl Pts',(136.64657075335,-209.363973465165,14.2773379372076));
#25168=CARTESIAN_POINT('Ctrl Pts',(138.497260071169,-208.140453793306,13.1216968983942));
#25169=CARTESIAN_POINT('Ctrl Pts',(140.914378515077,-206.504262153928,11.0274797072174));
#25170=CARTESIAN_POINT('Ctrl Pts',(141.679048846267,-205.980033579842,10.2626502639426));
#25171=CARTESIAN_POINT('Ctrl Pts',(143.080866831829,-205.008762402486,8.55915648524147));
#25172=CARTESIAN_POINT('Ctrl Pts',(143.717851327756,-204.561968106359,7.62021633376245));
#25173=CARTESIAN_POINT('Ctrl Pts',(144.775897909994,-203.814520750128,5.60723443384185));
#25174=CARTESIAN_POINT('Ctrl Pts',(145.197945099354,-203.513339264161,4.53064652501084));
#25175=CARTESIAN_POINT('Ctrl Pts',(145.767257174916,-203.105955734851,2.30184157443625));
#25176=CARTESIAN_POINT('Ctrl Pts',(145.914358443575,-203.,1.14953772934859));
#25177=CARTESIAN_POINT('Ctrl Pts',(145.914358443575,-203.,-5.55111512312578E-16));
#25178=CARTESIAN_POINT('',(258.115760998171,-203.,-2.32682891837997E-15));
#25179=CARTESIAN_POINT('',(258.115760998171,-203.,-2.32682891837997E-15));
#25180=CARTESIAN_POINT('Origin',(258.115760998171,-222.,0.));
#25181=CARTESIAN_POINT('Origin',(163.11576099817,-222.,0.));
#25182=CARTESIAN_POINT('',(121.453694879983,-207.,-1.8369702010623E-15));
#25183=CARTESIAN_POINT('Ctrl Pts',(121.453694879983,-207.,5.55111512312578E-16));
#25184=CARTESIAN_POINT('Ctrl Pts',(121.453694879983,-207.,0.907353133092068));
#25185=CARTESIAN_POINT('Ctrl Pts',(121.312112526369,-207.083231650701,1.80198099765884));
#25186=CARTESIAN_POINT('Ctrl Pts',(120.784107112644,-207.391641455618,3.5146797882098));
#25187=CARTESIAN_POINT('Ctrl Pts',(120.397755245695,-207.616671164825,4.33279938877936));
#25188=CARTESIAN_POINT('Ctrl Pts',(118.970528778436,-208.439967174701,6.61351349009191));
#25189=CARTESIAN_POINT('Ctrl Pts',(117.651916050567,-209.18968749672,7.90128916914638));
#25190=CARTESIAN_POINT('Ctrl Pts',(114.642831125276,-210.85711562393,10.1640207575769));
#25191=CARTESIAN_POINT('Ctrl Pts',(112.759779424709,-211.873400908832,11.1431178977762));
#25192=CARTESIAN_POINT('Ctrl Pts',(108.75053729299,-213.958936505348,12.7302152622124));
#25193=CARTESIAN_POINT('Ctrl Pts',(106.622299465224,-215.02926865615,13.3316141536719));
#25194=CARTESIAN_POINT('Ctrl Pts',(100.060775208621,-218.200471522578,14.6920280995398));
#25195=CARTESIAN_POINT('Ctrl Pts',(95.4525107000109,-220.249930762303,15.));
#25196=CARTESIAN_POINT('Ctrl Pts',(88.0210425552756,-223.302593927956,15.));
#25197=CARTESIAN_POINT('Ctrl Pts',(84.6790306087128,-224.594675453913,14.8289890919114));
#25198=CARTESIAN_POINT('Ctrl Pts',(77.8141827696673,-227.064438929898,14.1768373375443));
#25199=CARTESIAN_POINT('Ctrl Pts',(74.2912554085806,-228.242073248777,13.6964791866782));
#25200=CARTESIAN_POINT('Ctrl Pts',(67.2345931481628,-230.419495002038,12.4767593682344));
#25201=CARTESIAN_POINT('Ctrl Pts',(63.7008186732762,-231.41933527847,11.7385985584428));
#25202=CARTESIAN_POINT('Ctrl Pts',(56.8008352730486,-233.208850905064,10.0439158689026));
#25203=CARTESIAN_POINT('Ctrl Pts',(53.4336788142811,-233.998786023356,9.09152888694572));
#25204=CARTESIAN_POINT('Ctrl Pts',(48.5152345428215,-235.051962812042,7.4250013775077));
#25205=CARTESIAN_POINT('Ctrl Pts',(46.6209703458263,-235.43570474664,6.72770406164338));
#25206=CARTESIAN_POINT('Ctrl Pts',(43.8696416840566,-235.958313851502,5.51005073346341));
#25207=CARTESIAN_POINT('Ctrl Pts',(42.9682669434626,-236.123872251653,5.075737390253));
#25208=CARTESIAN_POINT('Ctrl Pts',(41.2574066533486,-236.428808311227,4.12993654891045));
#25209=CARTESIAN_POINT('Ctrl Pts',(40.4462113162161,-236.568461801527,3.62163429304668));
#25210=CARTESIAN_POINT('Ctrl Pts',(39.2605592418267,-236.767462602177,2.65913427303629));
#25211=CARTESIAN_POINT('Ctrl Pts',(38.7825283359309,-236.846042324477,2.20487590415701));
#25212=CARTESIAN_POINT('Ctrl Pts',(38.2440350776008,-236.933380610508,1.43553363474373));
#25213=CARTESIAN_POINT('Ctrl Pts',(38.0943087821406,-236.957453393979,1.16408998649961));
#25214=CARTESIAN_POINT('Ctrl Pts',(37.8864347500152,-236.990778602197,0.597557056254765));
#25215=CARTESIAN_POINT('Ctrl Pts',(37.8285606387555,-237.,0.302365587737163));
#25216=CARTESIAN_POINT('Ctrl Pts',(37.8285606387555,-237.,-0.302365587737163));
#25217=CARTESIAN_POINT('Ctrl Pts',(37.8864347500152,-236.990778602197,-0.597557056254765));
#25218=CARTESIAN_POINT('Ctrl Pts',(38.0943087821406,-236.957453393979,-1.16408998649961));
#25219=CARTESIAN_POINT('Ctrl Pts',(38.2440350776008,-236.933380610508,-1.43553363474373));
#25220=CARTESIAN_POINT('Ctrl Pts',(38.7825283359309,-236.846042324477,-2.20487590415701));
#25221=CARTESIAN_POINT('Ctrl Pts',(39.2605592418267,-236.767462602177,-2.65913427303629));
#25222=CARTESIAN_POINT('Ctrl Pts',(40.4462113162161,-236.568461801527,-3.62163429304668));
#25223=CARTESIAN_POINT('Ctrl Pts',(41.2574066533486,-236.428808311227,-4.12993654891045));
#25224=CARTESIAN_POINT('Ctrl Pts',(42.9682669434626,-236.123872251653,-5.075737390253));
#25225=CARTESIAN_POINT('Ctrl Pts',(43.8696416840566,-235.958313851502,-5.51005073346341));
#25226=CARTESIAN_POINT('Ctrl Pts',(46.6209703458263,-235.43570474664,-6.72770406164338));
#25227=CARTESIAN_POINT('Ctrl Pts',(48.5152345428215,-235.051962812042,-7.4250013775077));
#25228=CARTESIAN_POINT('Ctrl Pts',(53.4336788142811,-233.998786023356,-9.09152888694572));
#25229=CARTESIAN_POINT('Ctrl Pts',(56.8008352730486,-233.208850905064,-10.0439158689026));
#25230=CARTESIAN_POINT('Ctrl Pts',(63.7008186732762,-231.41933527847,-11.7385985584428));
#25231=CARTESIAN_POINT('Ctrl Pts',(67.2345931481628,-230.419495002038,-12.4767593682344));
#25232=CARTESIAN_POINT('Ctrl Pts',(74.2912554085806,-228.242073248777,-13.6964791866782));
#25233=CARTESIAN_POINT('Ctrl Pts',(77.8141827696673,-227.064438929898,-14.1768373375443));
#25234=CARTESIAN_POINT('Ctrl Pts',(84.6790306087128,-224.594675453913,-14.8289890919114));
#25235=CARTESIAN_POINT('Ctrl Pts',(88.0210425552756,-223.302593927956,-15.));
#25236=CARTESIAN_POINT('Ctrl Pts',(95.4525107000109,-220.249930762303,-15.));
#25237=CARTESIAN_POINT('Ctrl Pts',(100.060775208621,-218.200471522578,-14.6920280995398));
#25238=CARTESIAN_POINT('Ctrl Pts',(106.622299465224,-215.02926865615,-13.3316141536719));
#25239=CARTESIAN_POINT('Ctrl Pts',(108.75053729299,-213.958936505348,-12.7302152622124));
#25240=CARTESIAN_POINT('Ctrl Pts',(112.759779424709,-211.873400908832,-11.1431178977762));
#25241=CARTESIAN_POINT('Ctrl Pts',(114.642831125276,-210.85711562393,-10.1640207575769));
#25242=CARTESIAN_POINT('Ctrl Pts',(117.651916050567,-209.18968749672,-7.90128916914638));
#25243=CARTESIAN_POINT('Ctrl Pts',(118.970528778436,-208.439967174701,-6.61351349009191));
#25244=CARTESIAN_POINT('Ctrl Pts',(120.397755245695,-207.616671164825,-4.33279938877936));
#25245=CARTESIAN_POINT('Ctrl Pts',(120.784107112644,-207.391641455618,-3.5146797882098));
#25246=CARTESIAN_POINT('Ctrl Pts',(121.312112526369,-207.083231650701,-1.80198099765884));
#25247=CARTESIAN_POINT('Ctrl Pts',(121.453694879983,-207.,-0.907353133092065));
#25248=CARTESIAN_POINT('Ctrl Pts',(121.453694879983,-207.,2.77555756156289E-15));
#25249=CARTESIAN_POINT('',(263.115760998171,-207.,1.83697019872103E-15));
#25250=CARTESIAN_POINT('',(163.11576099817,-207.,1.83697019872103E-15));
#25251=CARTESIAN_POINT('Origin',(263.115760998171,-222.,0.));
#25252=CARTESIAN_POINT('Origin',(163.11576099817,222.,0.));
#25253=CARTESIAN_POINT('',(121.453694879983,207.,1.8369702010623E-15));
#25254=CARTESIAN_POINT('Ctrl Pts',(37.8285606387552,237.,6.76542155630955E-15));
#25255=CARTESIAN_POINT('Ctrl Pts',(37.8285606387552,237.,0.302365587737165));
#25256=CARTESIAN_POINT('Ctrl Pts',(37.8864347500152,236.990778602197,0.59755705625476));
#25257=CARTESIAN_POINT('Ctrl Pts',(38.0943087821406,236.957453393979,1.16408998649961));
#25258=CARTESIAN_POINT('Ctrl Pts',(38.2440350776008,236.933380610508,1.43553363474373));
#25259=CARTESIAN_POINT('Ctrl Pts',(38.7825283359309,236.846042324477,2.20487590415701));
#25260=CARTESIAN_POINT('Ctrl Pts',(39.2605592418267,236.767462602177,2.65913427303628));
#25261=CARTESIAN_POINT('Ctrl Pts',(40.4462113162161,236.568461801527,3.62163429304667));
#25262=CARTESIAN_POINT('Ctrl Pts',(41.2574066533486,236.428808311227,4.12993654891044));
#25263=CARTESIAN_POINT('Ctrl Pts',(42.9682669434626,236.123872251653,5.07573739025299));
#25264=CARTESIAN_POINT('Ctrl Pts',(43.8696416840566,235.958313851502,5.51005073346341));
#25265=CARTESIAN_POINT('Ctrl Pts',(46.6209703458263,235.43570474664,6.72770406164338));
#25266=CARTESIAN_POINT('Ctrl Pts',(48.5152345428215,235.051962812042,7.4250013775077));
#25267=CARTESIAN_POINT('Ctrl Pts',(53.4336788142811,233.998786023356,9.09152888694572));
#25268=CARTESIAN_POINT('Ctrl Pts',(56.8008352730486,233.208850905064,10.0439158689026));
#25269=CARTESIAN_POINT('Ctrl Pts',(63.7008186732762,231.41933527847,11.7385985584428));
#25270=CARTESIAN_POINT('Ctrl Pts',(67.2345931481628,230.419495002039,12.4767593682344));
#25271=CARTESIAN_POINT('Ctrl Pts',(74.2912554085806,228.242073248777,13.6964791866782));
#25272=CARTESIAN_POINT('Ctrl Pts',(77.8141827696673,227.064438929898,14.1768373375443));
#25273=CARTESIAN_POINT('Ctrl Pts',(84.6790306087128,224.594675453913,14.8289890919114));
#25274=CARTESIAN_POINT('Ctrl Pts',(88.0210425552756,223.302593927956,15.));
#25275=CARTESIAN_POINT('Ctrl Pts',(95.4525107000109,220.249930762303,15.));
#25276=CARTESIAN_POINT('Ctrl Pts',(100.060775208621,218.200471522578,14.6920280995398));
#25277=CARTESIAN_POINT('Ctrl Pts',(106.622299465224,215.02926865615,13.3316141536719));
#25278=CARTESIAN_POINT('Ctrl Pts',(108.75053729299,213.958936505348,12.7302152622124));
#25279=CARTESIAN_POINT('Ctrl Pts',(112.759779424709,211.873400908832,11.1431178977762));
#25280=CARTESIAN_POINT('Ctrl Pts',(114.642831125276,210.85711562393,10.1640207575769));
#25281=CARTESIAN_POINT('Ctrl Pts',(117.651916050567,209.18968749672,7.90128916914638));
#25282=CARTESIAN_POINT('Ctrl Pts',(118.970528778436,208.439967174701,6.6135134900919));
#25283=CARTESIAN_POINT('Ctrl Pts',(120.397755245695,207.616671164825,4.33279938877936));
#25284=CARTESIAN_POINT('Ctrl Pts',(120.784107112644,207.391641455618,3.5146797882098));
#25285=CARTESIAN_POINT('Ctrl Pts',(121.312112526369,207.083231650701,1.80198099765883));
#25286=CARTESIAN_POINT('Ctrl Pts',(121.453694879983,207.,0.907353133092066));
#25287=CARTESIAN_POINT('Ctrl Pts',(121.453694879983,207.,-0.907353133092066));
#25288=CARTESIAN_POINT('Ctrl Pts',(121.312112526369,207.083231650701,-1.80198099765884));
#25289=CARTESIAN_POINT('Ctrl Pts',(120.784107112644,207.391641455618,-3.5146797882098));
#25290=CARTESIAN_POINT('Ctrl Pts',(120.397755245695,207.616671164825,-4.33279938877936));
#25291=CARTESIAN_POINT('Ctrl Pts',(118.970528778436,208.439967174701,-6.6135134900919));
#25292=CARTESIAN_POINT('Ctrl Pts',(117.651916050567,209.18968749672,-7.90128916914638));
#25293=CARTESIAN_POINT('Ctrl Pts',(114.642831125276,210.85711562393,-10.1640207575769));
#25294=CARTESIAN_POINT('Ctrl Pts',(112.759779424709,211.873400908832,-11.1431178977762));
#25295=CARTESIAN_POINT('Ctrl Pts',(108.75053729299,213.958936505348,-12.7302152622124));
#25296=CARTESIAN_POINT('Ctrl Pts',(106.622299465224,215.02926865615,-13.3316141536719));
#25297=CARTESIAN_POINT('Ctrl Pts',(100.060775208621,218.200471522578,-14.6920280995398));
#25298=CARTESIAN_POINT('Ctrl Pts',(95.4525107000109,220.249930762303,-15.));
#25299=CARTESIAN_POINT('Ctrl Pts',(88.0210425552756,223.302593927956,-15.));
#25300=CARTESIAN_POINT('Ctrl Pts',(84.6790306087128,224.594675453913,-14.8289890919114));
#25301=CARTESIAN_POINT('Ctrl Pts',(77.8141827696673,227.064438929898,-14.1768373375443));
#25302=CARTESIAN_POINT('Ctrl Pts',(74.2912554085806,228.242073248777,-13.6964791866782));
#25303=CARTESIAN_POINT('Ctrl Pts',(67.2345931481628,230.419495002038,-12.4767593682344));
#25304=CARTESIAN_POINT('Ctrl Pts',(63.7008186732762,231.41933527847,-11.7385985584428));
#25305=CARTESIAN_POINT('Ctrl Pts',(56.8008352730486,233.208850905064,-10.0439158689026));
#25306=CARTESIAN_POINT('Ctrl Pts',(53.4336788142811,233.998786023356,-9.09152888694572));
#25307=CARTESIAN_POINT('Ctrl Pts',(48.5152345428215,235.051962812042,-7.4250013775077));
#25308=CARTESIAN_POINT('Ctrl Pts',(46.6209703458263,235.43570474664,-6.72770406164338));
#25309=CARTESIAN_POINT('Ctrl Pts',(43.8696416840566,235.958313851502,-5.51005073346341));
#25310=CARTESIAN_POINT('Ctrl Pts',(42.9682669434626,236.123872251653,-5.07573739025299));
#25311=CARTESIAN_POINT('Ctrl Pts',(41.2574066533486,236.428808311227,-4.12993654891044));
#25312=CARTESIAN_POINT('Ctrl Pts',(40.4462113162161,236.568461801527,-3.62163429304667));
#25313=CARTESIAN_POINT('Ctrl Pts',(39.2605592418267,236.767462602177,-2.65913427303628));
#25314=CARTESIAN_POINT('Ctrl Pts',(38.7825283359309,236.846042324477,-2.20487590415701));
#25315=CARTESIAN_POINT('Ctrl Pts',(38.2440350776008,236.933380610508,-1.43553363474373));
#25316=CARTESIAN_POINT('Ctrl Pts',(38.0943087821406,236.957453393979,-1.16408998649961));
#25317=CARTESIAN_POINT('Ctrl Pts',(37.8864347500152,236.990778602197,-0.597557056254762));
#25318=CARTESIAN_POINT('Ctrl Pts',(37.8285606387552,237.,-0.302365587737161));
#25319=CARTESIAN_POINT('Ctrl Pts',(37.8285606387552,237.,0.));
#25320=CARTESIAN_POINT('',(263.11576099817,207.,-1.83697019872103E-15));
#25321=CARTESIAN_POINT('',(163.11576099817,207.,-1.83697019872103E-15));
#25322=CARTESIAN_POINT('Origin',(263.11576099817,222.,0.));
#25323=CARTESIAN_POINT('Origin',(0.,0.,-65.));
#25324=CARTESIAN_POINT('',(-25.,-3.06161699786838E-15,-35.));
#25325=CARTESIAN_POINT('',(-25.,-3.06161699786838E-15,-65.));
#25326=CARTESIAN_POINT('Origin',(0.,0.,-35.));
#25327=CARTESIAN_POINT('Origin',(0.,267.,35.));
#25328=CARTESIAN_POINT('',(-2.5,267.,45.));
#25329=CARTESIAN_POINT('Origin',(0.,267.,45.));
#25330=CARTESIAN_POINT('',(-2.5,267.,55.));
#25331=CARTESIAN_POINT('',(-2.5,267.,35.));
#25332=CARTESIAN_POINT('Origin',(0.,267.,55.));
#25333=CARTESIAN_POINT('Origin',(108.598683701239,243.916637190574,35.));
#25334=CARTESIAN_POINT('',(106.098683701239,243.916637190574,45.));
#25335=CARTESIAN_POINT('Origin',(108.598683701239,243.916637190574,45.));
#25336=CARTESIAN_POINT('',(106.098683701239,243.916637190574,55.));
#25337=CARTESIAN_POINT('',(106.098683701239,243.916637190574,35.));
#25338=CARTESIAN_POINT('Origin',(108.598683701239,243.916637190574,55.));
#25339=CARTESIAN_POINT('Origin',(198.419668402464,178.657871897815,35.));
#25340=CARTESIAN_POINT('',(195.919668402464,178.657871897815,45.));
#25341=CARTESIAN_POINT('Origin',(198.419668402464,178.657871897815,45.));
#25342=CARTESIAN_POINT('',(195.919668402464,178.657871897815,55.));
#25343=CARTESIAN_POINT('',(195.919668402464,178.657871897815,35.));
#25344=CARTESIAN_POINT('Origin',(198.419668402464,178.657871897815,55.));
#25345=CARTESIAN_POINT('Origin',(253.932089850806,82.507537498111,35.));
#25346=CARTESIAN_POINT('',(251.432089850806,82.507537498111,45.));
#25347=CARTESIAN_POINT('Origin',(253.932089850806,82.507537498111,45.));
#25348=CARTESIAN_POINT('',(251.432089850806,82.507537498111,55.));
#25349=CARTESIAN_POINT('',(251.432089850806,82.507537498111,35.));
#25350=CARTESIAN_POINT('Origin',(253.932089850806,82.507537498111,55.));
#25351=CARTESIAN_POINT('Origin',(265.537346063329,-27.9090996924634,35.));
#25352=CARTESIAN_POINT('',(263.037346063329,-27.9090996924634,45.));
#25353=CARTESIAN_POINT('Origin',(265.537346063329,-27.9090996924634,45.));
#25354=CARTESIAN_POINT('',(263.037346063329,-27.9090996924634,55.));
#25355=CARTESIAN_POINT('',(263.037346063329,-27.9090996924634,35.));
#25356=CARTESIAN_POINT('Origin',(265.537346063329,-27.9090996924634,55.));
#25357=CARTESIAN_POINT('Origin',(231.228782810445,-133.5,35.));
#25358=CARTESIAN_POINT('',(228.728782810445,-133.5,45.));
#25359=CARTESIAN_POINT('Origin',(231.228782810445,-133.5,45.));
#25360=CARTESIAN_POINT('',(228.728782810445,-133.5,55.));
#25361=CARTESIAN_POINT('',(228.728782810445,-133.5,35.));
#25362=CARTESIAN_POINT('Origin',(231.228782810445,-133.5,55.));
#25363=CARTESIAN_POINT('Origin',(156.93866236209,-216.007537498111,35.));
#25364=CARTESIAN_POINT('',(154.43866236209,-216.007537498111,45.));
#25365=CARTESIAN_POINT('Origin',(156.93866236209,-216.007537498111,45.));
#25366=CARTESIAN_POINT('',(154.43866236209,-216.007537498111,55.));
#25367=CARTESIAN_POINT('',(154.43866236209,-216.007537498111,35.));
#25368=CARTESIAN_POINT('Origin',(156.93866236209,-216.007537498111,55.));
#25369=CARTESIAN_POINT('Origin',(55.5124214483419,-261.165409395926,35.));
#25370=CARTESIAN_POINT('',(53.0124214483419,-261.165409395926,45.));
#25371=CARTESIAN_POINT('Origin',(55.5124214483419,-261.165409395926,45.));
#25372=CARTESIAN_POINT('',(53.0124214483419,-261.165409395926,55.));
#25373=CARTESIAN_POINT('',(53.0124214483419,-261.165409395926,35.));
#25374=CARTESIAN_POINT('Origin',(55.5124214483419,-261.165409395926,55.));
#25375=CARTESIAN_POINT('Origin',(-55.5124214483417,-261.165409395926,35.));
#25376=CARTESIAN_POINT('',(-58.0124214483417,-261.165409395926,45.));
#25377=CARTESIAN_POINT('Origin',(-55.5124214483417,-261.165409395926,45.));
#25378=CARTESIAN_POINT('',(-58.0124214483417,-261.165409395926,55.));
#25379=CARTESIAN_POINT('',(-58.0124214483417,-261.165409395926,35.));
#25380=CARTESIAN_POINT('Origin',(-55.5124214483417,-261.165409395926,55.));
#25381=CARTESIAN_POINT('Origin',(-156.93866236209,-216.007537498111,35.));
#25382=CARTESIAN_POINT('',(-159.43866236209,-216.007537498111,45.));
#25383=CARTESIAN_POINT('Origin',(-156.93866236209,-216.007537498111,45.));
#25384=CARTESIAN_POINT('',(-159.43866236209,-216.007537498111,55.));
#25385=CARTESIAN_POINT('',(-159.43866236209,-216.007537498111,35.));
#25386=CARTESIAN_POINT('Origin',(-156.93866236209,-216.007537498111,55.));
#25387=CARTESIAN_POINT('Origin',(-231.228782810445,-133.5,35.));
#25388=CARTESIAN_POINT('',(-233.728782810445,-133.5,45.));
#25389=CARTESIAN_POINT('Origin',(-231.228782810445,-133.5,45.));
#25390=CARTESIAN_POINT('',(-233.728782810445,-133.5,55.));
#25391=CARTESIAN_POINT('',(-233.728782810445,-133.5,35.));
#25392=CARTESIAN_POINT('Origin',(-231.228782810445,-133.5,55.));
#25393=CARTESIAN_POINT('Origin',(-265.537346063329,-27.9090996924637,35.));
#25394=CARTESIAN_POINT('',(-268.037346063329,-27.9090996924637,45.));
#25395=CARTESIAN_POINT('Origin',(-265.537346063329,-27.9090996924637,45.));
#25396=CARTESIAN_POINT('',(-268.037346063329,-27.9090996924637,55.));
#25397=CARTESIAN_POINT('',(-268.037346063329,-27.9090996924637,35.));
#25398=CARTESIAN_POINT('Origin',(-265.537346063329,-27.9090996924637,55.));
#25399=CARTESIAN_POINT('Origin',(-253.932089850806,82.5075374981109,35.));
#25400=CARTESIAN_POINT('',(-256.432089850806,82.5075374981109,45.));
#25401=CARTESIAN_POINT('Origin',(-253.932089850806,82.5075374981109,45.));
#25402=CARTESIAN_POINT('',(-256.432089850806,82.5075374981109,55.));
#25403=CARTESIAN_POINT('',(-256.432089850806,82.5075374981109,35.));
#25404=CARTESIAN_POINT('Origin',(-253.932089850806,82.5075374981109,55.));
#25405=CARTESIAN_POINT('Origin',(-198.419668402464,178.657871897815,35.));
#25406=CARTESIAN_POINT('',(-200.919668402464,178.657871897815,45.));
#25407=CARTESIAN_POINT('Origin',(-198.419668402464,178.657871897815,45.));
#25408=CARTESIAN_POINT('',(-200.919668402464,178.657871897815,55.));
#25409=CARTESIAN_POINT('',(-200.919668402464,178.657871897815,35.));
#25410=CARTESIAN_POINT('Origin',(-198.419668402464,178.657871897815,55.));
#25411=CARTESIAN_POINT('Origin',(-108.598683701239,243.916637190575,35.));
#25412=CARTESIAN_POINT('',(-111.098683701239,243.916637190575,45.));
#25413=CARTESIAN_POINT('Origin',(-108.598683701239,243.916637190575,45.));
#25414=CARTESIAN_POINT('',(-111.098683701239,243.916637190575,55.));
#25415=CARTESIAN_POINT('',(-111.098683701239,243.916637190575,35.));
#25416=CARTESIAN_POINT('Origin',(-108.598683701239,243.916637190575,55.));
#25417=CARTESIAN_POINT('Origin',(0.,0.,55.));
#25418=CARTESIAN_POINT('',(250.,-3.06161699786838E-14,45.));
#25419=CARTESIAN_POINT('',(250.,-3.06161699786838E-14,55.));
#25420=CARTESIAN_POINT('Origin',(0.,0.,45.));
#25421=CARTESIAN_POINT('Origin',(0.,0.,45.));
#25422=CARTESIAN_POINT('',(-275.,-3.36777869765522E-14,55.));
#25423=CARTESIAN_POINT('Origin',(0.,0.,55.));
#25424=CARTESIAN_POINT('',(-275.,-3.36777869765522E-14,45.));
#25425=CARTESIAN_POINT('',(-275.,-3.36777869765522E-14,45.));
#25426=CARTESIAN_POINT('Origin',(0.,0.,45.));
#25427=CARTESIAN_POINT('Origin',(0.,0.,-733.822509939086));
#25428=CARTESIAN_POINT('',(-240.,-2.93915231795365E-14,-45.));
#25429=CARTESIAN_POINT('Origin',(0.,0.,-45.));
#25430=CARTESIAN_POINT('',(-240.,-2.93915231795365E-14,55.));
#25431=CARTESIAN_POINT('',(-240.,-2.93915231795365E-14,-733.822509939086));
#25432=CARTESIAN_POINT('Origin',(0.,0.,55.));
#25433=CARTESIAN_POINT('Origin',(0.,0.,-45.));
#25434=CARTESIAN_POINT('',(42.0243552790815,46.1933668131508,-45.));
#25435=CARTESIAN_POINT('',(42.0243552790815,46.193366813151,-45.));
#25436=CARTESIAN_POINT('',(61.0168067860623,13.2974758427732,-45.));
#25437=CARTESIAN_POINT('',(61.0168067860623,13.2974758427731,-45.));
#25438=CARTESIAN_POINT('',(61.885047674397,8.37343707771113,-45.));
#25439=CARTESIAN_POINT('',(61.885047674397,8.37343707771212,-45.));
#25440=CARTESIAN_POINT('',(61.885047674397,8.37343707771212,-45.));
#25441=CARTESIAN_POINT('',(55.289038487168,-29.0343899078532,-45.));
#25442=CARTESIAN_POINT('',(55.289038487168,-29.0343899078532,-45.));
#25443=CARTESIAN_POINT('',(52.7890384871678,-33.3645169267754,-45.));
#25444=CARTESIAN_POINT('',(52.789038487168,-33.3645169267754,-45.));
#25445=CARTESIAN_POINT('',(52.789038487168,-33.3645169267754,-45.));
#25446=CARTESIAN_POINT('',(23.6909146109103,-57.7807419392945,-45.));
#25447=CARTESIAN_POINT('',(23.6909146109103,-57.7807419392945,-45.));
#25448=CARTESIAN_POINT('',(18.9924515069803,-59.4908426559229,-45.));
#25449=CARTESIAN_POINT('',(18.9924515069808,-59.4908426559229,-45.));
#25450=CARTESIAN_POINT('',(18.9924515069808,-59.4908426559229,-45.));
#25451=CARTESIAN_POINT('',(-18.99245150698,-59.4908426559232,-45.));
#25452=CARTESIAN_POINT('',(-18.99245150698,-59.4908426559232,-45.));
#25453=CARTESIAN_POINT('',(-23.6909146109095,-57.7807419392947,-45.));
#25454=CARTESIAN_POINT('',(-23.6909146109095,-57.7807419392948,-45.));
#25455=CARTESIAN_POINT('',(-23.6909146109095,-57.7807419392948,-45.));
#25456=CARTESIAN_POINT('',(-52.7890384871676,-33.3645169267762,-45.));
#25457=CARTESIAN_POINT('',(-52.7890384871676,-33.3645169267762,-45.));
#25458=CARTESIAN_POINT('',(-55.2890384871676,-29.0343899078537,-45.));
#25459=CARTESIAN_POINT('',(-55.2890384871676,-29.034389907854,-45.));
#25460=CARTESIAN_POINT('',(-55.2890384871676,-29.034389907854,-45.));
#25461=CARTESIAN_POINT('',(-61.8850476743971,8.3734370777113,-45.));
#25462=CARTESIAN_POINT('',(-61.8850476743971,8.3734370777113,-45.));
#25463=CARTESIAN_POINT('',(-61.0168067860623,13.2974758427723,-45.));
#25464=CARTESIAN_POINT('',(-61.0168067860625,13.2974758427723,-45.));
#25465=CARTESIAN_POINT('',(-61.0168067860625,13.2974758427723,-45.));
#25466=CARTESIAN_POINT('',(-42.0243552790822,46.1933668131505,-45.));
#25467=CARTESIAN_POINT('',(-42.0243552790822,46.1933668131505,-45.));
#25468=CARTESIAN_POINT('',(-38.194133063487,49.4073048615832,-45.));
#25469=CARTESIAN_POINT('',(-38.1941330634873,49.4073048615832,-45.));
#25470=CARTESIAN_POINT('',(-38.1941330634873,49.4073048615832,-45.));
#25471=CARTESIAN_POINT('',(-2.5,62.3989068346297,-45.));
#25472=CARTESIAN_POINT('',(-2.5,62.3989068346297,-45.));
#25473=CARTESIAN_POINT('',(2.5,62.3989068346295,-45.));
#25474=CARTESIAN_POINT('',(2.5,62.3989068346297,-45.));
#25475=CARTESIAN_POINT('',(2.5,62.3989068346297,-45.));
#25476=CARTESIAN_POINT('',(38.1941330634866,49.4073048615837,-45.));
#25477=CARTESIAN_POINT('',(38.1941330634866,49.4073048615837,-45.));
#25478=CARTESIAN_POINT('',(42.0243552790815,46.193366813151,-45.));
#25479=CARTESIAN_POINT('Origin',(0.,0.,55.));
#25480=CARTESIAN_POINT('Origin',(0.,0.,45.));
#25481=CARTESIAN_POINT('Origin',(0.,0.,-55.));
#25482=CARTESIAN_POINT('Origin',(263.115760998171,202.,-20.));
#25483=CARTESIAN_POINT('',(263.115760998171,197.,-20.));
#25484=CARTESIAN_POINT('',(263.115760998171,202.,-25.));
#25485=CARTESIAN_POINT('Origin',(263.115760998171,202.,-20.));
#25486=CARTESIAN_POINT('',(263.11576099817,242.,-25.));
#25487=CARTESIAN_POINT('',(263.115760998171,202.,-25.));
#25488=CARTESIAN_POINT('',(263.11576099817,247.,-20.));
#25489=CARTESIAN_POINT('Origin',(263.11576099817,242.,-20.));
#25490=CARTESIAN_POINT('',(263.11576099817,247.,20.));
#25491=CARTESIAN_POINT('',(263.11576099817,247.,20.));
#25492=CARTESIAN_POINT('',(263.11576099817,242.,25.));
#25493=CARTESIAN_POINT('Origin',(263.11576099817,242.,20.));
#25494=CARTESIAN_POINT('',(263.115760998171,202.,25.));
#25495=CARTESIAN_POINT('',(263.115760998171,202.,25.));
#25496=CARTESIAN_POINT('',(263.115760998171,197.,20.));
#25497=CARTESIAN_POINT('Origin',(263.115760998171,202.,20.));
#25498=CARTESIAN_POINT('',(263.115760998171,197.,20.));
#25499=CARTESIAN_POINT('Origin',(258.115760998171,202.,-20.));
#25500=CARTESIAN_POINT('',(258.115760998171,197.,-20.));
#25501=CARTESIAN_POINT('',(258.115760998171,202.,-25.));
#25502=CARTESIAN_POINT('Origin',(258.115760998171,202.,-20.));
#25503=CARTESIAN_POINT('',(258.115760998171,197.,20.));
#25504=CARTESIAN_POINT('',(258.115760998171,197.,20.));
#25505=CARTESIAN_POINT('',(258.115760998171,202.,25.));
#25506=CARTESIAN_POINT('Origin',(258.115760998171,202.,20.));
#25507=CARTESIAN_POINT('',(258.11576099817,242.,25.));
#25508=CARTESIAN_POINT('',(258.115760998171,202.,25.));
#25509=CARTESIAN_POINT('',(258.11576099817,247.,20.));
#25510=CARTESIAN_POINT('Origin',(258.11576099817,242.,20.));
#25511=CARTESIAN_POINT('',(258.11576099817,247.,-20.));
#25512=CARTESIAN_POINT('',(258.11576099817,247.,20.));
#25513=CARTESIAN_POINT('',(258.11576099817,242.,-25.));
#25514=CARTESIAN_POINT('Origin',(258.11576099817,242.,-20.));
#25515=CARTESIAN_POINT('',(258.115760998171,202.,-25.));
#25516=CARTESIAN_POINT('Origin',(263.115760998171,202.,-20.));
#25517=CARTESIAN_POINT('',(263.115760998171,202.,-25.));
#25518=CARTESIAN_POINT('',(263.115760998171,197.,-20.));
#25519=CARTESIAN_POINT('Origin',(263.115760998171,202.,-25.));
#25520=CARTESIAN_POINT('',(263.11576099817,242.,-25.));
#25521=CARTESIAN_POINT('Origin',(263.11576099817,242.,-20.));
#25522=CARTESIAN_POINT('',(263.11576099817,247.,-20.));
#25523=CARTESIAN_POINT('Origin',(263.11576099817,247.,20.));
#25524=CARTESIAN_POINT('',(263.11576099817,247.,20.));
#25525=CARTESIAN_POINT('Origin',(263.11576099817,242.,20.));
#25526=CARTESIAN_POINT('',(263.11576099817,242.,25.));
#25527=CARTESIAN_POINT('Origin',(263.115760998171,202.,25.));
#25528=CARTESIAN_POINT('',(263.115760998171,202.,25.));
#25529=CARTESIAN_POINT('Origin',(263.115760998171,202.,20.));
#25530=CARTESIAN_POINT('',(263.115760998171,197.,20.));
#25531=CARTESIAN_POINT('Origin',(263.115760998171,197.,20.));
#25532=CARTESIAN_POINT('Origin',(263.115760998171,-242.,-20.));
#25533=CARTESIAN_POINT('',(263.115760998171,-247.,-20.));
#25534=CARTESIAN_POINT('',(263.115760998171,-242.,-25.));
#25535=CARTESIAN_POINT('Origin',(263.115760998171,-242.,-20.));
#25536=CARTESIAN_POINT('',(263.115760998171,-202.,-25.));
#25537=CARTESIAN_POINT('',(263.115760998171,-202.,-25.));
#25538=CARTESIAN_POINT('',(263.115760998171,-197.,-20.));
#25539=CARTESIAN_POINT('Origin',(263.115760998171,-202.,-20.));
#25540=CARTESIAN_POINT('',(263.115760998171,-197.,20.));
#25541=CARTESIAN_POINT('',(263.115760998171,-197.,20.));
#25542=CARTESIAN_POINT('',(263.115760998171,-202.,25.));
#25543=CARTESIAN_POINT('Origin',(263.115760998171,-202.,20.));
#25544=CARTESIAN_POINT('',(263.115760998171,-242.,25.));
#25545=CARTESIAN_POINT('',(263.115760998171,-202.,25.));
#25546=CARTESIAN_POINT('',(263.115760998171,-247.,20.));
#25547=CARTESIAN_POINT('Origin',(263.115760998171,-242.,20.));
#25548=CARTESIAN_POINT('',(263.115760998171,-247.,20.));
#25549=CARTESIAN_POINT('Origin',(258.115760998171,-242.,-20.));
#25550=CARTESIAN_POINT('',(258.115760998171,-247.,-20.));
#25551=CARTESIAN_POINT('',(258.115760998171,-242.,-25.));
#25552=CARTESIAN_POINT('Origin',(258.115760998171,-242.,-20.));
#25553=CARTESIAN_POINT('',(258.115760998171,-247.,20.));
#25554=CARTESIAN_POINT('',(258.115760998171,-247.,20.));
#25555=CARTESIAN_POINT('',(258.115760998171,-242.,25.));
#25556=CARTESIAN_POINT('Origin',(258.115760998171,-242.,20.));
#25557=CARTESIAN_POINT('',(258.115760998171,-202.,25.));
#25558=CARTESIAN_POINT('',(258.115760998171,-202.,25.));
#25559=CARTESIAN_POINT('',(258.115760998171,-197.,20.));
#25560=CARTESIAN_POINT('Origin',(258.115760998171,-202.,20.));
#25561=CARTESIAN_POINT('',(258.115760998171,-197.,-20.));
#25562=CARTESIAN_POINT('',(258.115760998171,-197.,20.));
#25563=CARTESIAN_POINT('',(258.115760998171,-202.,-25.));
#25564=CARTESIAN_POINT('Origin',(258.115760998171,-202.,-20.));
#25565=CARTESIAN_POINT('',(258.115760998171,-202.,-25.));
#25566=CARTESIAN_POINT('Origin',(263.115760998171,-242.,-20.));
#25567=CARTESIAN_POINT('',(263.115760998171,-242.,-25.));
#25568=CARTESIAN_POINT('',(263.115760998171,-247.,-20.));
#25569=CARTESIAN_POINT('Origin',(263.115760998171,-202.,-25.));
#25570=CARTESIAN_POINT('',(263.115760998171,-202.,-25.));
#25571=CARTESIAN_POINT('Origin',(263.115760998171,-202.,-20.));
#25572=CARTESIAN_POINT('',(263.115760998171,-197.,-20.));
#25573=CARTESIAN_POINT('Origin',(263.115760998171,-197.,20.));
#25574=CARTESIAN_POINT('',(263.115760998171,-197.,20.));
#25575=CARTESIAN_POINT('Origin',(263.115760998171,-202.,20.));
#25576=CARTESIAN_POINT('',(263.115760998171,-202.,25.));
#25577=CARTESIAN_POINT('Origin',(263.115760998171,-202.,25.));
#25578=CARTESIAN_POINT('',(263.115760998171,-242.,25.));
#25579=CARTESIAN_POINT('Origin',(263.115760998171,-242.,20.));
#25580=CARTESIAN_POINT('',(263.115760998171,-247.,20.));
#25581=CARTESIAN_POINT('Origin',(263.115760998171,-247.,20.));
#25582=CARTESIAN_POINT('Origin',(0.,0.,-35.));
#25583=CARTESIAN_POINT('Origin',(2.5,0.,0.));
#25584=CARTESIAN_POINT('',(2.5,30.,-35.));
#25585=CARTESIAN_POINT('Origin',(-2.5,0.,0.));
#25586=CARTESIAN_POINT('',(-2.5,30.,-35.));
#25587=CARTESIAN_POINT('Origin',(2.5,30.,-35.));
#25588=CARTESIAN_POINT('Origin',(1.91511110779744,1.60696902421635,0.));
#25589=CARTESIAN_POINT('',(-17.3685171827988,24.5883023177857,-35.));
#25590=CARTESIAN_POINT('Origin',(-1.91511110779744,-1.60696902421635,0.));
#25591=CARTESIAN_POINT('',(-21.1987393983937,21.374364269353,-35.));
#25592=CARTESIAN_POINT('Origin',(-17.3685171827988,24.5883023177857,-35.));
#25593=CARTESIAN_POINT('Origin',(0.434120444167318,2.46201938253052,0.));
#25594=CARTESIAN_POINT('',(-29.1101121461989,7.67146471253834,-35.));
#25595=CARTESIAN_POINT('Origin',(-0.434120444167318,-2.46201938253052,0.));
#25596=CARTESIAN_POINT('',(-29.9783530345336,2.7474259474773,-35.));
#25597=CARTESIAN_POINT('Origin',(-29.1101121461989,7.67146471253834,-35.));
#25598=CARTESIAN_POINT('Origin',(-1.25000000000001,2.16506350946109,0.));
#25599=CARTESIAN_POINT('',(-27.2307621135331,-12.834936490539,-35.));
#25600=CARTESIAN_POINT('Origin',(1.25000000000001,-2.16506350946109,0.));
#25601=CARTESIAN_POINT('',(-24.7307621135331,-17.1650635094612,-35.));
#25602=CARTESIAN_POINT('Origin',(-27.2307621135331,-12.834936490539,-35.));
#25603=CARTESIAN_POINT('Origin',(-2.34923155196478,0.855050358314158,0.));
#25604=CARTESIAN_POINT('',(-12.6098358517347,-27.3357282652632,-35.));
#25605=CARTESIAN_POINT('Origin',(2.34923155196478,-0.855050358314158,0.));
#25606=CARTESIAN_POINT('',(-7.91137274780512,-29.0458289818915,-35.));
#25607=CARTESIAN_POINT('Origin',(-12.6098358517347,-27.3357282652632,-35.));
#25608=CARTESIAN_POINT('Origin',(-2.34923155196477,-0.855050358314189,0.));
#25609=CARTESIAN_POINT('',(7.91137274780551,-29.0458289818914,-35.));
#25610=CARTESIAN_POINT('Origin',(2.34923155196477,0.855050358314189,0.));
#25611=CARTESIAN_POINT('',(12.609835851735,-27.335728265263,-35.));
#25612=CARTESIAN_POINT('Origin',(7.91137274780551,-29.0458289818914,-35.));
#25613=CARTESIAN_POINT('Origin',(-1.24999999999998,-2.16506350946111,0.));
#25614=CARTESIAN_POINT('',(24.7307621135333,-17.1650635094609,-35.));
#25615=CARTESIAN_POINT('Origin',(1.24999999999998,2.16506350946111,0.));
#25616=CARTESIAN_POINT('',(27.2307621135333,-12.8349364905386,-35.));
#25617=CARTESIAN_POINT('Origin',(24.7307621135333,-17.1650635094609,-35.));
#25618=CARTESIAN_POINT('Origin',(0.434120444167351,-2.46201938253052,0.));
#25619=CARTESIAN_POINT('',(29.9783530345335,2.7474259474777,-35.));
#25620=CARTESIAN_POINT('Origin',(-0.434120444167351,2.46201938253052,0.));
#25621=CARTESIAN_POINT('',(29.1101121461988,7.67146471253873,-35.));
#25622=CARTESIAN_POINT('Origin',(29.9783530345335,2.7474259474777,-35.));
#25623=CARTESIAN_POINT('Origin',(1.91511110779746,-1.60696902421633,0.));
#25624=CARTESIAN_POINT('',(21.1987393983934,21.3743642693533,-35.));
#25625=CARTESIAN_POINT('Origin',(-1.91511110779746,1.60696902421633,0.));
#25626=CARTESIAN_POINT('',(17.3685171827984,24.5883023177859,-35.));
#25627=CARTESIAN_POINT('Origin',(21.1987393983934,21.3743642693533,-35.));
#39943=UNCERTAINTY_MEASURE_WITH_UNIT(LENGTH_MEASURE(0.01),#39960,
'DISTANCE_ACCURACY_VALUE',
'Maximum model space distance between geometric entities at asserted c
onnectivities');
#39950=UNCERTAINTY_MEASURE_WITH_UNIT(LENGTH_MEASURE(0.01),#39960,
'DISTANCE_ACCURACY_VALUE',
'Maximum model space distance between geometric entities at asserted c
onnectivities');
#39952=(
GEOMETRIC_REPRESENTATION_CONTEXT(3)
GLOBAL_UNCERTAINTY_ASSIGNED_CONTEXT((#39943))
GLOBAL_UNIT_ASSIGNED_CONTEXT((#39960,#39962,#39963))
REPRESENTATION_CONTEXT('','3D')
);
#39959=(
GEOMETRIC_REPRESENTATION_CONTEXT(3)
GLOBAL_UNCERTAINTY_ASSIGNED_CONTEXT((#39950))
GLOBAL_UNIT_ASSIGNED_CONTEXT((#39960,#39962,#39963))
REPRESENTATION_CONTEXT('','3D')
);
#39960=(
LENGTH_UNIT()
NAMED_UNIT(*)
SI_UNIT(.MILLI.,.METRE.)
);
#39962=(
NAMED_UNIT(*)
PLANE_ANGLE_UNIT()
SI_UNIT($,.RADIAN.)
);
#39963=(
NAMED_UNIT(*)
SI_UNIT($,.STERADIAN.)
SOLID_ANGLE_UNIT()
);
#39965=SHAPE_DEFINITION_REPRESENTATION(#39973,#40002);
#39973=PRODUCT_DEFINITION_SHAPE('',$,#40011);
#40002=SHAPE_REPRESENTATION('',(#18350),#39952);
#40009=PRODUCT_DEFINITION_CONTEXT('part definition',#40035,'design');
#40011=PRODUCT_DEFINITION('Main Cover','Main Cover',#40019,#40009);
#40019=PRODUCT_DEFINITION_FORMATION('',$,#40038);
#40035=APPLICATION_CONTEXT(
'Core Data for Automotive Mechanical Design Process');
#40036=PRODUCT_CONTEXT('part definition',#40035,'mechanical');
#40038=PRODUCT('Main Cover','Main Cover',$,(#40036));
#40046=PRESENTATION_STYLE_ASSIGNMENT((#40048));
#40048=SURFACE_STYLE_USAGE(.BOTH.,#40050);
#40050=SURFACE_SIDE_STYLE('',(#40052));
#40052=SURFACE_STYLE_FILL_AREA(#40054);
#40054=FILL_AREA_STYLE('Opaque(202,209,238)',(#40056));
#40056=FILL_AREA_STYLE_COLOUR('Opaque(202,209,238)',#40058);
#40058=COLOUR_RGB('Opaque(202,209,238)', 0.66274510, 0.83137255, 0.94901961);
ENDSEC;
END-ISO-10303-21;
